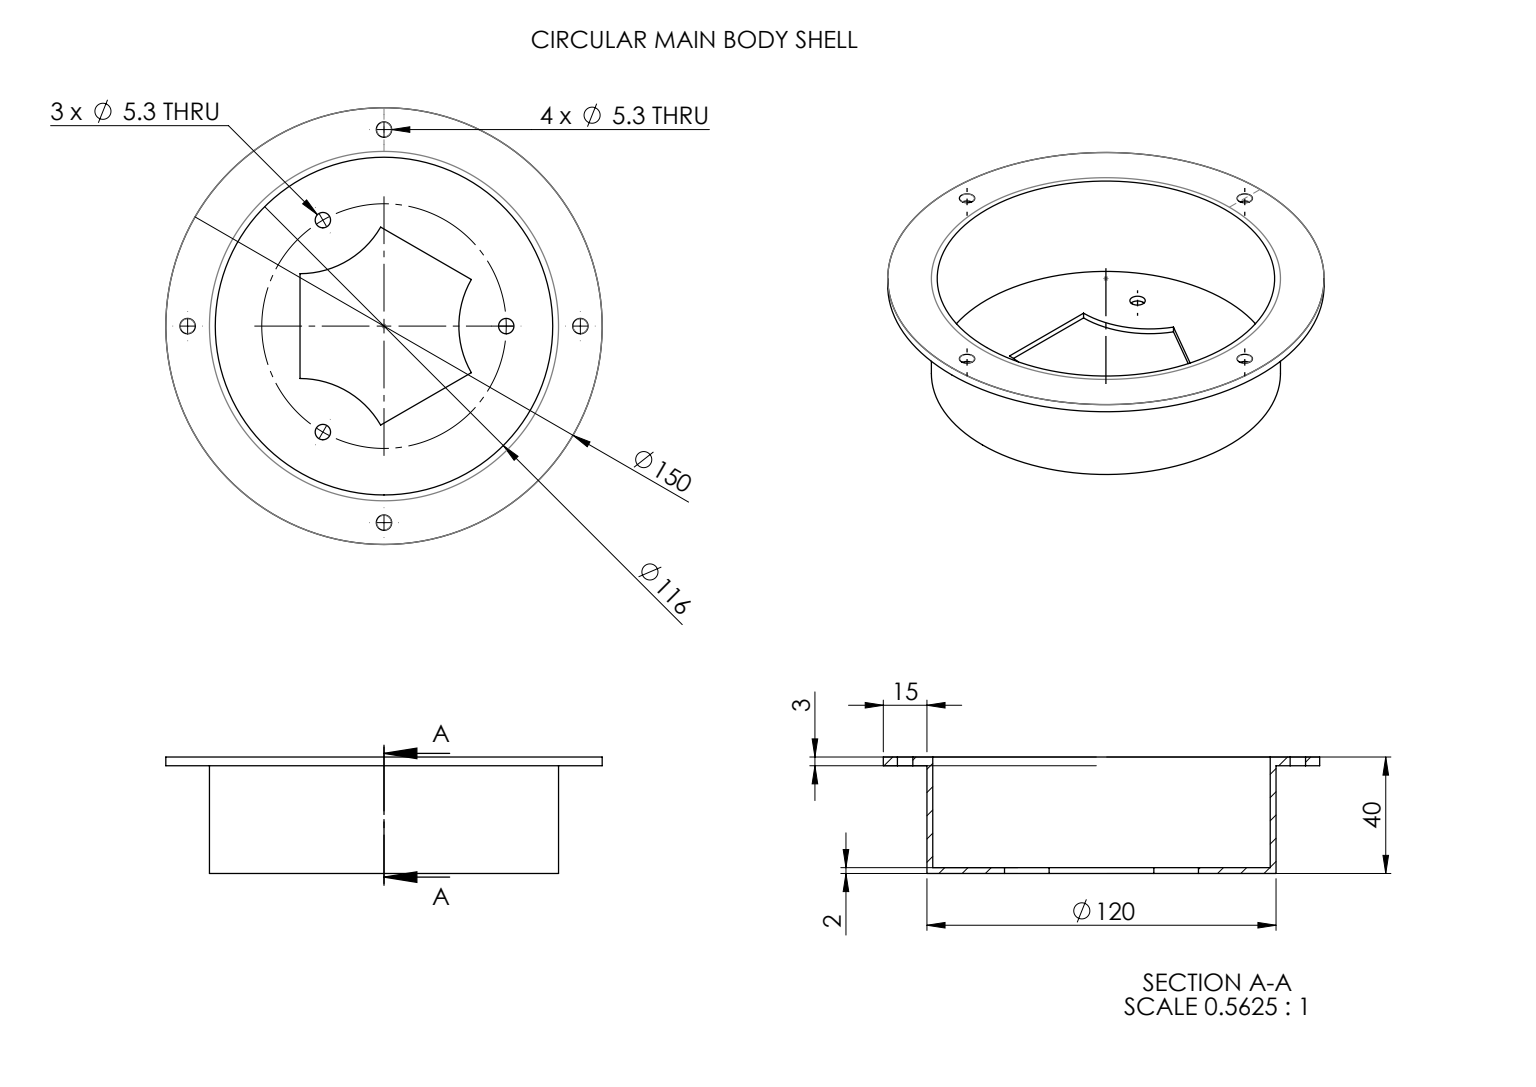
ISO-10303-21;
HEADER;
FILE_DESCRIPTION (('STEP AP214'),
    '1' );
FILE_NAME ('Circular Main Body Shell.step',
    '2026-10-08T13:56:24',
    ( '' ),
    ( '' ),
    'SwSTEP 2.0',
    'SolidWorks 2026',
    '' );
FILE_SCHEMA (( 'AUTOMOTIVE_DESIGN' ));
ENDSEC;

DATA;
#6=VERTEX_POINT ( 'NONE', #1075 ) ;
#10=FACE_OUTER_BOUND ( 'NONE', #8516, .T. ) ;
#19=CYLINDRICAL_SURFACE ( 'NONE', #13536, 2.649999999999992806 ) ;
#21=ADVANCED_FACE ( 'NONE', ( #13423 ), #15876, .F. ) ;
#33=DIRECTION ( 'NONE',  ( 0.000000000000000000, 1.000000000000000000, 0.000000000000000000 ) ) ;
#56=ORIENTED_EDGE ( 'NONE', *, *, #13519, .T. ) ;
#59=VERTEX_POINT ( 'NONE', #6499 ) ;
#76=DIRECTION ( 'NONE',  ( 0.000000000000000000, 1.000000000000000000, 0.000000000000000000 ) ) ;
#81=VECTOR ( 'NONE', #2135, 1000.000000000000000 ) ;
#82=CYLINDRICAL_SURFACE ( 'NONE', #8761, 60.00000000000000000 ) ;
#83=EDGE_CURVE ( 'NONE', #1457, #7914, #2680, .T. ) ;
#86=EDGE_CURVE ( 'NONE', #59, #10154, #4028, .T. ) ;
#101=VECTOR ( 'NONE', #11182, 1000.000000000000000 ) ;
#111=ORIENTED_EDGE ( 'NONE', *, *, #9988, .F. ) ;
#132=DIRECTION ( 'NONE',  ( -0.000000000000000000, -1.000000000000000000, -0.000000000000000000 ) ) ;
#138=VERTEX_POINT ( 'NONE', #361 ) ;
#140=DIRECTION ( 'NONE',  ( 0.000000000000000000, 0.000000000000000000, -1.000000000000000000 ) ) ;
#144=( GEOMETRIC_REPRESENTATION_CONTEXT ( 3 ) GLOBAL_UNCERTAINTY_ASSIGNED_CONTEXT ( ( #8076 ) ) GLOBAL_UNIT_ASSIGNED_CONTEXT ( ( #8304, #5944, #13354 ) ) REPRESENTATION_CONTEXT ( 'NONE', 'WORKASPACE' ) );
#151=DIRECTION ( 'NONE',  ( 0.000000000000000000, 1.000000000000000000, 0.000000000000000000 ) ) ;
#167=VECTOR ( 'NONE', #2072, 1000.000000000000000 ) ;
#187=AXIS2_PLACEMENT_3D ( 'NONE', #15569, #9111, #5544 ) ;
#226=EDGE_CURVE ( 'NONE', #3694, #59, #13994, .T. ) ;
#237=CARTESIAN_POINT ( 'NONE',  ( 0.000000000000000000, 37.00000000000000000, 0.000000000000000000 ) ) ;
#246=ORIENTED_EDGE ( 'NONE', *, *, #2734, .T. ) ;
#248=ORIENTED_EDGE ( 'NONE', *, *, #7361, .F. ) ;
#256=AXIS2_PLACEMENT_3D ( 'NONE', #544, #2863, #5079 ) ;
#267=ORIENTED_EDGE ( 'NONE', *, *, #8923, .F. ) ;
#295=PRODUCT_DEFINITION_CONTEXT ( 'detailed design', #4442, 'design' ) ;
#312=EDGE_CURVE ( 'NONE', #2273, #15957, #6128, .T. ) ;
#325=ORIENTED_EDGE ( 'NONE', *, *, #13615, .F. ) ;
#345=AXIS2_PLACEMENT_3D ( 'NONE', #12427, #14786, #2573 ) ;
#361=CARTESIAN_POINT ( 'NONE',  ( 67.49999999999931788, 40.00000000000000000, 2.650000000000013678 ) ) ;
#364=ADVANCED_FACE ( 'NONE', ( #4243 ), #462, .T. ) ;
#368=CARTESIAN_POINT ( 'NONE',  ( 0.000000000000000000, 40.00000000000000000, 0.000000000000000000 ) ) ;
#377=ORIENTED_EDGE ( 'NONE', *, *, #15710, .F. ) ;
#382=DIRECTION ( 'NONE',  ( -0.000000000000000000, -1.000000000000000000, -0.000000000000000000 ) ) ;
#387=CIRCLE ( 'NONE', #3230, 2.649999999999985700 ) ;
#406=DIRECTION ( 'NONE',  ( -0.000000000000000000, -1.000000000000000000, -0.000000000000000000 ) ) ;
#415=PLANE ( 'NONE',  #1616 ) ;
#434=VERTEX_POINT ( 'NONE', #14346 ) ;
#447=DIRECTION ( 'NONE',  ( 0.000000000000000000, 0.000000000000000000, 1.000000000000000000 ) ) ;
#452=AXIS2_PLACEMENT_3D ( 'NONE', #5371, #14093, #447 ) ;
#460=EDGE_LOOP ( 'NONE', ( #1578, #12472, #3436, #12198 ) ) ;
#462=CYLINDRICAL_SURFACE ( 'NONE', #5357, 75.00000000000001421 ) ;
#515=CARTESIAN_POINT ( 'NONE',  ( 0.000000000000000000, 37.00000000000000000, 75.00000000000001421 ) ) ;
#544=CARTESIAN_POINT ( 'NONE',  ( -67.50000000000000000, 40.00000000000000000, -7.070249711157346244E-13 ) ) ;
#558=EDGE_LOOP ( 'NONE', ( #4178, #10902, #2223, #13257 ) ) ;
#573=DIRECTION ( 'NONE',  ( 0.000000000000000000, 1.000000000000000000, 0.000000000000000000 ) ) ;
#584=DIRECTION ( 'NONE',  ( 0.000000000000000000, 1.000000000000000000, 0.000000000000000000 ) ) ;
#615=VERTEX_POINT ( 'NONE', #3712 ) ;
#631=CARTESIAN_POINT ( 'NONE',  ( 2.143131898507869826E-15, 37.00000000000000000, -67.50000000000000000 ) ) ;
#642=EDGE_LOOP ( 'NONE', ( #4159, #10843 ) ) ;
#646=DIRECTION ( 'NONE',  ( -0.000000000000000000, -1.000000000000000000, -0.000000000000000000 ) ) ;
#660=VECTOR ( 'NONE', #7753, 1000.000000000000000 ) ;
#674=CIRCLE ( 'NONE', #6869, 2.649999999999985700 ) ;
#675=ORIENTED_EDGE ( 'NONE', *, *, #4801, .F. ) ;
#688=EDGE_CURVE ( 'NONE', #4101, #6399, #11429, .T. ) ;
#691=( NAMED_UNIT ( * ) SI_UNIT ( $, .STERADIAN. ) SOLID_ANGLE_UNIT ( ) );
#694=AXIS2_PLACEMENT_3D ( 'NONE', #3412, #1145, #4634 ) ;
#706=DIRECTION ( 'NONE',  ( 0.000000000000000000, 0.000000000000000000, 1.000000000000000000 ) ) ;
#731=CIRCLE ( 'NONE', #9748, 32.00000000000000000 ) ;
#738=EDGE_LOOP ( 'NONE', ( #9185, #775, #5500, #912 ) ) ;
#739=VERTEX_POINT ( 'NONE', #11389 ) ;
#759=VECTOR ( 'NONE', #12567, 1000.000000000000000 ) ;
#760=ORIENTED_EDGE ( 'NONE', *, *, #7226, .T. ) ;
#775=ORIENTED_EDGE ( 'NONE', *, *, #5162, .T. ) ;
#783=FACE_BOUND ( 'NONE', #9056, .T. ) ;
#792=ORIENTED_EDGE ( 'NONE', *, *, #4767, .T. ) ;
#825=CARTESIAN_POINT ( 'NONE',  ( 0.000000000000000000, 37.00000000000000000, 0.000000000000000000 ) ) ;
#826=AXIS2_PLACEMENT_3D ( 'NONE', #2213, #7167, #7316 ) ;
#833=ADVANCED_FACE ( 'NONE', ( #10189, #4033, #2825, #6724, #1611 ), #415, .T. ) ;
#865=VERTEX_POINT ( 'NONE', #5510 ) ;
#881=DIRECTION ( 'NONE',  ( -0.000000000000000000, -1.000000000000000000, -0.000000000000000000 ) ) ;
#896=PLANE ( 'NONE',  #9190 ) ;
#911=( GEOMETRIC_REPRESENTATION_CONTEXT ( 3 ) GLOBAL_UNCERTAINTY_ASSIGNED_CONTEXT ( ( #10140 ) ) GLOBAL_UNIT_ASSIGNED_CONTEXT ( ( #15799, #6830, #4795 ) ) REPRESENTATION_CONTEXT ( 'NONE', 'WORKASPACE' ) );
#912=ORIENTED_EDGE ( 'NONE', *, *, #2834, .T. ) ;
#945=EDGE_LOOP ( 'NONE', ( #10035, #9827 ) ) ;
#946=VERTEX_POINT ( 'NONE', #1706 ) ;
#953=EDGE_CURVE ( 'NONE', #7835, #12023, #11561, .T. ) ;
#956=ADVANCED_FACE ( 'NONE', ( #10366 ), #15296, .F. ) ;
#975=DIRECTION ( 'NONE',  ( -0.000000000000000000, -1.000000000000000000, -0.000000000000000000 ) ) ;
#976=AXIS2_PLACEMENT_3D ( 'NONE', #15540, #4455, #14550 ) ;
#986=AXIS2_PLACEMENT_3D ( 'NONE', #11840, #10645, #6771 ) ;
#989=ORIENTED_EDGE ( 'NONE', *, *, #8609, .T. ) ;
#1007=ORIENTED_EDGE ( 'NONE', *, *, #15616, .T. ) ;
#1038=DIRECTION ( 'NONE',  ( 0.000000000000000000, 1.000000000000000000, 0.000000000000000000 ) ) ;
#1044=LINE ( 'NONE', #14705, #13288 ) ;
#1056=ORIENTED_EDGE ( 'NONE', *, *, #14475, .T. ) ;
#1062=ORIENTED_EDGE ( 'NONE', *, *, #11599, .T. ) ;
#1070=CARTESIAN_POINT ( 'NONE',  ( -1.154700538379255903, 0.000000000000000000, 34.00000000000000000 ) ) ;
#1075=CARTESIAN_POINT ( 'NONE',  ( 42.02221399786069611, -1.230770033143087371E-15, -2.649999999999878231 ) ) ;
#1080=SURFACE_SIDE_STYLE ('',( #10941 ) ) ;
#1120=LINE ( 'NONE', #3465, #2794 ) ;
#1134=CARTESIAN_POINT ( 'NONE',  ( 57.73502691896258199, -20.00000000000000000, 2.081668171172168513E-14 ) ) ;
#1145=DIRECTION ( 'NONE',  ( 0.000000000000000000, 1.000000000000000000, 0.000000000000000000 ) ) ;
#1150=ORIENTED_EDGE ( 'NONE', *, *, #5943, .T. ) ;
#1154=FILL_AREA_STYLE ('',( #15648 ) ) ;
#1161=EDGE_CURVE ( 'NONE', #13011, #10876, #5502, .T. ) ;
#1169=VERTEX_POINT ( 'NONE', #13399 ) ;
#1225=AXIS2_PLACEMENT_3D ( 'NONE', #6934, #1826, #1750 ) ;
#1235=ADVANCED_FACE ( 'NONE', ( #10 ), #1285, .F. ) ;
#1263=FACE_BOUND ( 'NONE', #7017, .T. ) ;
#1275=VERTEX_POINT ( 'NONE', #12264 ) ;
#1281=ORIENTED_EDGE ( 'NONE', *, *, #8662, .T. ) ;
#1285=CYLINDRICAL_SURFACE ( 'NONE', #6526, 2.649999999999992806 ) ;
#1356=DIRECTION ( 'NONE',  ( -0.000000000000000000, -1.000000000000000000, -0.000000000000000000 ) ) ;
#1371=EDGE_LOOP ( 'NONE', ( #10340, #15637, #15181, #9864 ) ) ;
#1374=ORIENTED_EDGE ( 'NONE', *, *, #4282, .F. ) ;
#1383=EDGE_CURVE ( 'NONE', #138, #615, #4026, .T. ) ;
#1387=ORIENTED_EDGE ( 'NONE', *, *, #5738, .T. ) ;
#1457=VERTEX_POINT ( 'NONE', #5415 ) ;
#1471=CARTESIAN_POINT ( 'NONE',  ( 67.49999999999931788, 40.00000000000000000, 2.081668171172168513E-14 ) ) ;
#1478=CIRCLE ( 'NONE', #4839, 60.00000000000000000 ) ;
#1494=CARTESIAN_POINT ( 'NONE',  ( 67.49999999999931788, 37.00000000000000000, -2.649999999999964828 ) ) ;
#1526=EDGE_LOOP ( 'NONE', ( #5441, #6855, #1062, #15045 ) ) ;
#1531=LINE ( 'NONE', #13549, #15735 ) ;
#1533=DIRECTION ( 'NONE',  ( -0.000000000000000000, -1.000000000000000000, -0.000000000000000000 ) ) ;
#1555=ADVANCED_FACE ( 'NONE', ( #7105 ), #2081, .F. ) ;
#1578=ORIENTED_EDGE ( 'NONE', *, *, #15530, .F. ) ;
#1590=CIRCLE ( 'NONE', #826, 2.649999999999985700 ) ;
#1611=FACE_BOUND ( 'NONE', #4354, .T. ) ;
#1616=AXIS2_PLACEMENT_3D ( 'NONE', #5338, #10277, #15205 ) ;
#1618=AXIS2_PLACEMENT_3D ( 'NONE', #10717, #15416, #6844 ) ;
#1635=DIRECTION ( 'NONE',  ( -0.000000000000000000, -1.000000000000000000, -0.000000000000000000 ) ) ;
#1654=VERTEX_POINT ( 'NONE', #7262 ) ;
#1662=AXIS2_PLACEMENT_3D ( 'NONE', #13941, #5063, #2795 ) ;
#1671=ORIENTED_EDGE ( 'NONE', *, *, #6597, .T. ) ;
#1673=( GEOMETRIC_REPRESENTATION_CONTEXT ( 3 ) GLOBAL_UNCERTAINTY_ASSIGNED_CONTEXT ( ( #6941 ) ) GLOBAL_UNIT_ASSIGNED_CONTEXT ( ( #8215, #13115, #691 ) ) REPRESENTATION_CONTEXT ( 'NONE', 'WORKASPACE' ) );
#1706=CARTESIAN_POINT ( 'NONE',  ( -28.86751345948145442, 1.999999999999994893, -18.00000000000001066 ) ) ;
#1713=CIRCLE ( 'NONE', #1979, 57.99999999999999289 ) ;
#1717=EDGE_LOOP ( 'NONE', ( #3204, #14325, #8748, #11994 ) ) ;
#1718=AXIS2_PLACEMENT_3D ( 'NONE', #2231, #7261, #4667 ) ;
#1732=EDGE_CURVE ( 'NONE', #1275, #10154, #13943, .T. ) ;
#1750=DIRECTION ( 'NONE',  ( 0.000000000000000000, 0.000000000000000000, 1.000000000000000000 ) ) ;
#1779=CARTESIAN_POINT ( 'NONE',  ( 0.000000000000000000, 2.000000000000001776, -57.99999999999999289 ) ) ;
#1792=PRODUCT_CONTEXT ( 'NONE', #13090, 'mechanical' ) ;
#1798=ORIENTED_EDGE ( 'NONE', *, *, #688, .F. ) ;
#1811=EDGE_CURVE ( 'NONE', #1275, #3694, #5749, .T. ) ;
#1826=DIRECTION ( 'NONE',  ( 0.000000000000000000, 1.000000000000000000, 0.000000000000000000 ) ) ;
#1838=DIRECTION ( 'NONE',  ( 0.000000000000000000, 0.000000000000000000, -1.000000000000000000 ) ) ;
#1846=CARTESIAN_POINT ( 'NONE',  ( -21.01110699893060030, 2.000000000000000000, 36.39230484541324273 ) ) ;
#1851=EDGE_LOOP ( 'NONE', ( #10259, #13734, #246, #14447 ) ) ;
#1854=DIRECTION ( 'NONE',  ( 9.048317650695024227E-15, 0.000000000000000000, 1.000000000000000000 ) ) ;
#1863=SHAPE_DEFINITION_REPRESENTATION ( #4609, #14733 ) ;
#1889=EDGE_LOOP ( 'NONE', ( #3943, #12784, #12058, #10841 ) ) ;
#1902=PLANE ( 'NONE',  #13101 ) ;
#1931=VECTOR ( 'NONE', #6950, 1000.000000000000000 ) ;
#1933=ADVANCED_FACE ( 'NONE', ( #14354, #11835, #11910, #783, #3283, #4415 ), #5777, .T. ) ;
#1939=VECTOR ( 'NONE', #2696, 1000.000000000000227 ) ;
#1971=EDGE_CURVE ( 'NONE', #2273, #15878, #13430, .T. ) ;
#1979=AXIS2_PLACEMENT_3D ( 'NONE', #2128, #11091, #15945 ) ;
#1989=PRODUCT_DEFINITION_FORMATION_WITH_SPECIFIED_SOURCE ( 'ANY', '', #3575, .NOT_KNOWN. ) ;
#1992=DIRECTION ( 'NONE',  ( -0.000000000000000000, -1.000000000000000000, -0.000000000000000000 ) ) ;
#2010=DIRECTION ( 'NONE',  ( 0.000000000000000000, 0.000000000000000000, 1.000000000000000000 ) ) ;
#2016=ORIENTED_EDGE ( 'NONE', *, *, #6491, .F. ) ;
#2035=CIRCLE ( 'NONE', #4097, 2.649999999999985700 ) ;
#2040=DIRECTION ( 'NONE',  ( 0.000000000000000000, 0.000000000000000000, -1.000000000000000000 ) ) ;
#2044=EDGE_CURVE ( 'NONE', #7914, #615, #1590, .T. ) ;
#2067=FACE_OUTER_BOUND ( 'NONE', #12399, .T. ) ;
#2072=DIRECTION ( 'NONE',  ( -0.000000000000000000, -1.000000000000000000, -0.000000000000000000 ) ) ;
#2075=ORIENTED_EDGE ( 'NONE', *, *, #11616, .F. ) ;
#2078=CARTESIAN_POINT ( 'NONE',  ( 0.000000000000000000, 40.00000000000000000, -57.99999999999999289 ) ) ;
#2081=CYLINDRICAL_SURFACE ( 'NONE', #8849, 2.649999999999992806 ) ;
#2083=ADVANCED_FACE ( 'NONE', ( #12146 ), #6102, .F. ) ;
#2091=DIRECTION ( 'NONE',  ( 0.000000000000000000, 0.000000000000000000, -1.000000000000000000 ) ) ;
#2096=FACE_OUTER_BOUND ( 'NONE', #1526, .T. ) ;
#2128=CARTESIAN_POINT ( 'NONE',  ( 0.000000000000000000, 2.000000000000001776, 0.000000000000000000 ) ) ;
#2131=SURFACE_STYLE_USAGE ( .BOTH. , #1080 ) ;
#2134=CARTESIAN_POINT ( 'NONE',  ( -50.51988060489983212, 0.000000000000000000, 62.50099999999999767 ) ) ;
#2135=DIRECTION ( 'NONE',  ( -0.000000000000000000, -1.000000000000000000, -0.000000000000000000 ) ) ;
#2151=DIRECTION ( 'NONE',  ( -0.000000000000000000, -1.000000000000000000, -0.000000000000000000 ) ) ;
#2164=FACE_BOUND ( 'NONE', #10857, .T. ) ;
#2174=ORIENTED_EDGE ( 'NONE', *, *, #2044, .T. ) ;
#2198=CYLINDRICAL_SURFACE ( 'NONE', #694, 75.00000000000001421 ) ;
#2203=SURFACE_STYLE_FILL_AREA ( #14189 ) ;
#2213=CARTESIAN_POINT ( 'NONE',  ( 67.49999999999931788, 37.00000000000000000, 2.081668171172168513E-14 ) ) ;
#2220=VERTEX_POINT ( 'NONE', #14073 ) ;
#2223=ORIENTED_EDGE ( 'NONE', *, *, #7879, .T. ) ;
#2231=CARTESIAN_POINT ( 'NONE',  ( -21.01110699893060030, 2.000000000000000000, 36.39230484541324273 ) ) ;
#2234=VECTOR ( 'NONE', #10201, 1000.000000000000000 ) ;
#2235=DIRECTION ( 'NONE',  ( -0.000000000000000000, -1.000000000000000000, -0.000000000000000000 ) ) ;
#2250=LINE ( 'NONE', #8497, #12002 ) ;
#2273=VERTEX_POINT ( 'NONE', #5913 ) ;
#2274=CIRCLE ( 'NONE', #11563, 57.99999999999999289 ) ;
#2361=CARTESIAN_POINT ( 'NONE',  ( 42.02221399786069611, 0.000000000000000000, 1.075528555105620399E-13 ) ) ;
#2403=FACE_OUTER_BOUND ( 'NONE', #3347, .T. ) ;
#2484=DIRECTION ( 'NONE',  ( 0.000000000000000000, 0.000000000000000000, 1.000000000000000000 ) ) ;
#2502=AXIS2_PLACEMENT_3D ( 'NONE', #8052, #3348, #14421 ) ;
#2560=ORIENTED_EDGE ( 'NONE', *, *, #5738, .F. ) ;
#2571=DIRECTION ( 'NONE',  ( -0.000000000000000000, -1.000000000000000000, -0.000000000000000000 ) ) ;
#2573=DIRECTION ( 'NONE',  ( 0.000000000000000000, 0.000000000000000000, -1.000000000000000000 ) ) ;
#2596=EDGE_LOOP ( 'NONE', ( #9917, #6295, #11447, #4939 ) ) ;
#2617=DIRECTION ( 'NONE',  ( 0.000000000000000000, 0.000000000000000000, -1.000000000000000000 ) ) ;
#2668=CARTESIAN_POINT ( 'NONE',  ( 9.184850993605150311E-15, 37.00000000000000000, -75.00000000000001421 ) ) ;
#2673=DIRECTION ( 'NONE',  ( 0.000000000000000000, 0.000000000000000000, 1.000000000000000000 ) ) ;
#2676=DIRECTION ( 'NONE',  ( -0.000000000000000000, -1.000000000000000000, -0.000000000000000000 ) ) ;
#2680=LINE ( 'NONE', #15061, #6377 ) ;
#2685=CIRCLE ( 'NONE', #8936, 2.649999999999985700 ) ;
#2686=CIRCLE ( 'NONE', #10444, 2.649999999999985700 ) ;
#2696=DIRECTION ( 'NONE',  ( -0.8660254037844408170, -0.000000000000000000, -0.4999999999999961142 ) ) ;
#2702=ORIENTED_EDGE ( 'NONE', *, *, #8509, .T. ) ;
#2731=EDGE_CURVE ( 'NONE', #15878, #1169, #11203, .T. ) ;
#2734=EDGE_CURVE ( 'NONE', #615, #7914, #2686, .T. ) ;
#2745=ORIENTED_EDGE ( 'NONE', *, *, #6491, .T. ) ;
#2772=EDGE_CURVE ( 'NONE', #7134, #5346, #13221, .T. ) ;
#2792=AXIS2_PLACEMENT_3D ( 'NONE', #14224, #4368, #9302 ) ;
#2793=FACE_OUTER_BOUND ( 'NONE', #15403, .T. ) ;
#2794=VECTOR ( 'NONE', #975, 1000.000000000000000 ) ;
#2795=DIRECTION ( 'NONE',  ( 0.000000000000000000, 0.000000000000000000, 1.000000000000000000 ) ) ;
#2825=FACE_BOUND ( 'NONE', #13224, .T. ) ;
#2834=EDGE_CURVE ( 'NONE', #434, #10287, #5541, .T. ) ;
#2849=AXIS2_PLACEMENT_3D ( 'NONE', #10462, #4319, #9259 ) ;
#2863=DIRECTION ( 'NONE',  ( 0.000000000000000000, 1.000000000000000000, 0.000000000000000000 ) ) ;
#2924=EDGE_LOOP ( 'NONE', ( #7893, #9587, #3567, #3170 ) ) ;
#2973=CARTESIAN_POINT ( 'NONE',  ( 67.49999999999931788, 37.00000000000000000, 2.650000000000013678 ) ) ;
#2986=ORIENTED_EDGE ( 'NONE', *, *, #3942, .F. ) ;
#2996=DIRECTION ( 'NONE',  ( 0.4999999999999998890, 0.000000000000000000, 0.8660254037844387076 ) ) ;
#3012=VECTOR ( 'NONE', #7245, 1000.000000000000000 ) ;
#3032=CARTESIAN_POINT ( 'NONE',  ( -6.765421556309547668E-13, 40.00000000000000000, 67.49999999999930367 ) ) ;
#3035=EDGE_CURVE ( 'NONE', #5346, #10287, #3930, .T. ) ;
#3043=CIRCLE ( 'NONE', #14152, 75.00000000000001421 ) ;
#3044=CARTESIAN_POINT ( 'NONE',  ( 0.000000000000000000, 0.000000000000000000, 0.000000000000000000 ) ) ;
#3079=ORIENTED_EDGE ( 'NONE', *, *, #14190, .T. ) ;
#3087=CIRCLE ( 'NONE', #256, 2.649999999999992806 ) ;
#3100=ORIENTED_EDGE ( 'NONE', *, *, #5391, .T. ) ;
#3112=ORIENTED_EDGE ( 'NONE', *, *, #5162, .F. ) ;
#3120=FACE_OUTER_BOUND ( 'NONE', #4526, .T. ) ;
#3122=CARTESIAN_POINT ( 'NONE',  ( -28.86751345948126257, -20.00000000000000000, -50.00000000000000711 ) ) ;
#3125=LINE ( 'NONE', #10644, #10930 ) ;
#3145=DIRECTION ( 'NONE',  ( 0.000000000000000000, 1.000000000000000000, 0.000000000000000000 ) ) ;
#3170=ORIENTED_EDGE ( 'NONE', *, *, #7879, .F. ) ;
#3192=ORIENTED_EDGE ( 'NONE', *, *, #4801, .T. ) ;
#3200=DIRECTION ( 'NONE',  ( -0.000000000000000000, -1.000000000000000000, -0.000000000000000000 ) ) ;
#3204=ORIENTED_EDGE ( 'NONE', *, *, #8662, .F. ) ;
#3223=AXIS2_PLACEMENT_3D ( 'NONE', #11897, #11972, #4638 ) ;
#3227=PLANE ( 'NONE',  #6600 ) ;
#3230=AXIS2_PLACEMENT_3D ( 'NONE', #10329, #7502, #11515 ) ;
#3235=EDGE_CURVE ( 'NONE', #15957, #1169, #3125, .T. ) ;
#3254=ADVANCED_FACE ( 'NONE', ( #5867 ), #15574, .F. ) ;
#3268=SURFACE_STYLE_USAGE ( .BOTH. , #7154 ) ;
#3279=ADVANCED_FACE ( 'NONE', ( #2067 ), #1902, .F. ) ;
#3282=AXIS2_PLACEMENT_3D ( 'NONE', #11517, #7666, #12565 ) ;
#3283=FACE_BOUND ( 'NONE', #12989, .T. ) ;
#3286=DIRECTION ( 'NONE',  ( -0.000000000000000000, -1.000000000000000000, -0.000000000000000000 ) ) ;
#3333=EDGE_LOOP ( 'NONE', ( #12994, #325 ) ) ;
#3346=EDGE_CURVE ( 'NONE', #7037, #1654, #14509, .T. ) ;
#3347=EDGE_LOOP ( 'NONE', ( #5791, #8130, #7271, #13989 ) ) ;
#3348=DIRECTION ( 'NONE',  ( 0.000000000000000000, 1.000000000000000000, 0.000000000000000000 ) ) ;
#3361=DIRECTION ( 'NONE',  ( 0.000000000000000000, 0.000000000000000000, -1.000000000000000000 ) ) ;
#3391=ORIENTED_EDGE ( 'NONE', *, *, #83, .T. ) ;
#3412=CARTESIAN_POINT ( 'NONE',  ( 0.000000000000000000, 37.00000000000000000, 0.000000000000000000 ) ) ;
#3429=CARTESIAN_POINT ( 'NONE',  ( 0.000000000000000000, 40.00000000000000000, -57.99999999999999289 ) ) ;
#3436=ORIENTED_EDGE ( 'NONE', *, *, #3346, .T. ) ;
#3442=FACE_OUTER_BOUND ( 'NONE', #11276, .T. ) ;
#3465=CARTESIAN_POINT ( 'NONE',  ( 42.02221399786069611, 0.000000000000000000, -2.649999999999884892 ) ) ;
#3467=CARTESIAN_POINT ( 'NONE',  ( -21.01110699893060030, 0.000000000000000000, 36.39230484541324273 ) ) ;
#3480=EDGE_CURVE ( 'NONE', #11871, #12864, #13849, .T. ) ;
#3500=AXIS2_PLACEMENT_3D ( 'NONE', #5960, #2151, #8629 ) ;
#3527=VECTOR ( 'NONE', #1635, 1000.000000000000000 ) ;
#3548=AXIS2_PLACEMENT_3D ( 'NONE', #10049, #6414, #2673 ) ;
#3567=ORIENTED_EDGE ( 'NONE', *, *, #12620, .F. ) ;
#3575=PRODUCT ( 'Circular Main Body Shell', 'Circular Main Body Shell', '', ( #1792 ) ) ;
#3577=FACE_OUTER_BOUND ( 'NONE', #13494, .T. ) ;
#3608=FACE_BOUND ( 'NONE', #15163, .T. ) ;
#3665=ADVANCED_FACE ( 'NONE', ( #15396 ), #5528, .F. ) ;
#3678=ORIENTED_EDGE ( 'NONE', *, *, #7728, .T. ) ;
#3694=VERTEX_POINT ( 'NONE', #8048 ) ;
#3695=CARTESIAN_POINT ( 'NONE',  ( 79.38739406438118351, 1.999999999999998224, 12.50099999999964417 ) ) ;
#3705=DIRECTION ( 'NONE',  ( -0.000000000000000000, -1.000000000000000000, -0.000000000000000000 ) ) ;
#3712=CARTESIAN_POINT ( 'NONE',  ( 67.49999999999931788, 37.00000000000000000, 2.650000000000006573 ) ) ;
#3755=ADVANCED_FACE ( 'NONE', ( #3577 ), #2198, .T. ) ;
#3766=DIRECTION ( 'NONE',  ( 0.000000000000000000, -0.000000000000000000, 1.000000000000000000 ) ) ;
#3773=DIRECTION ( 'NONE',  ( 0.000000000000000000, 0.000000000000000000, 1.000000000000000000 ) ) ;
#3894=EDGE_LOOP ( 'NONE', ( #8906, #760 ) ) ;
#3924=ADVANCED_FACE ( 'NONE', ( #5112 ), #8837, .T. ) ;
#3930=LINE ( 'NONE', #12806, #4979 ) ;
#3937=ORIENTED_EDGE ( 'NONE', *, *, #7399, .F. ) ;
#3942=EDGE_CURVE ( 'NONE', #138, #1457, #7143, .T. ) ;
#3943=ORIENTED_EDGE ( 'NONE', *, *, #6047, .T. ) ;
#3995=EDGE_LOOP ( 'NONE', ( #1798, #13792, #7346, #5691 ) ) ;
#4004=CARTESIAN_POINT ( 'NONE',  ( -50.51988060489983212, 1.999999999999998224, 62.50099999999999767 ) ) ;
#4017=VECTOR ( 'NONE', #1356, 1000.000000000000000 ) ;
#4026=LINE ( 'NONE', #2973, #9618 ) ;
#4028=CIRCLE ( 'NONE', #12800, 60.00000000000000000 ) ;
#4033=FACE_BOUND ( 'NONE', #11763, .T. ) ;
#4038=ORIENTED_EDGE ( 'NONE', *, *, #3942, .T. ) ;
#4042=VERTEX_POINT ( 'NONE', #8037 ) ;
#4057=ORIENTED_EDGE ( 'NONE', *, *, #3235, .F. ) ;
#4097=AXIS2_PLACEMENT_3D ( 'NONE', #11691, #4188, #1838 ) ;
#4101=VERTEX_POINT ( 'NONE', #8943 ) ;
#4106=ORIENTED_EDGE ( 'NONE', *, *, #226, .F. ) ;
#4110=CIRCLE ( 'NONE', #5926, 57.99999999999999289 ) ;
#4154=CARTESIAN_POINT ( 'NONE',  ( 2.143131898507869826E-15, 37.00000000000000000, -67.50000000000000000 ) ) ;
#4159=ORIENTED_EDGE ( 'NONE', *, *, #12723, .F. ) ;
#4167=DIRECTION ( 'NONE',  ( -0.000000000000000000, -1.000000000000000000, -0.000000000000000000 ) ) ;
#4178=ORIENTED_EDGE ( 'NONE', *, *, #13550, .F. ) ;
#4187=DIRECTION ( 'NONE',  ( 0.000000000000000000, 0.000000000000000000, -1.000000000000000000 ) ) ;
#4188=DIRECTION ( 'NONE',  ( -0.000000000000000000, -1.000000000000000000, -0.000000000000000000 ) ) ;
#4209=CARTESIAN_POINT ( 'NONE',  ( -50.51988060489983212, 1.999999999999998224, 62.50099999999999767 ) ) ;
#4225=CARTESIAN_POINT ( 'NONE',  ( 42.02221399786069611, 2.000000000000000000, 1.075528555105620399E-13 ) ) ;
#4243=FACE_OUTER_BOUND ( 'NONE', #6518, .T. ) ;
#4279=DIRECTION ( 'NONE',  ( 8.673617379884035472E-16, 0.000000000000000000, 1.000000000000000000 ) ) ;
#4282=EDGE_CURVE ( 'NONE', #14880, #10728, #7157, .T. ) ;
#4319=DIRECTION ( 'NONE',  ( -0.000000000000000000, -1.000000000000000000, -0.000000000000000000 ) ) ;
#4323=ORIENTED_EDGE ( 'NONE', *, *, #15530, .T. ) ;
#4326=CARTESIAN_POINT ( 'NONE',  ( -1.154700538379235031, 1.999999999999998224, -34.00000000000000000 ) ) ;
#4354=EDGE_LOOP ( 'NONE', ( #2016, #3937, #6611, #9493, #248, #8433 ) ) ;
#4367=DIRECTION ( 'NONE',  ( -0.000000000000000000, -1.000000000000000000, -0.000000000000000000 ) ) ;
#4368=DIRECTION ( 'NONE',  ( -0.000000000000000000, -1.000000000000000000, -0.000000000000000000 ) ) ;
#4375=ORIENTED_EDGE ( 'NONE', *, *, #9521, .T. ) ;
#4385=FACE_OUTER_BOUND ( 'NONE', #14907, .T. ) ;
#4412=DIRECTION ( 'NONE',  ( 0.000000000000000000, 1.000000000000000000, 0.000000000000000000 ) ) ;
#4415=FACE_OUTER_BOUND ( 'NONE', #6444, .T. ) ;
#4442=APPLICATION_CONTEXT ( 'automotive_design' ) ;
#4444=FACE_BOUND ( 'NONE', #945, .T. ) ;
#4455=DIRECTION ( 'NONE',  ( -0.000000000000000000, -1.000000000000000000, -0.000000000000000000 ) ) ;
#4467=AXIS2_PLACEMENT_3D ( 'NONE', #11083, #8823, #14055 ) ;
#4498=EDGE_LOOP ( 'NONE', ( #14987, #11958 ) ) ;
#4513=CARTESIAN_POINT ( 'NONE',  ( 67.49999999999931788, 37.00000000000000000, 2.081668171172168513E-14 ) ) ;
#4519=FACE_BOUND ( 'NONE', #8353, .T. ) ;
#4526=EDGE_LOOP ( 'NONE', ( #14542, #13389, #13917, #11725 ) ) ;
#4538=VECTOR ( 'NONE', #14752, 1000.000000000000000 ) ;
#4545=ADVANCED_FACE ( 'NONE', ( #11286 ), #9040, .F. ) ;
#4566=PRESENTATION_STYLE_ASSIGNMENT (( #2131 ) ) ;
#4579=ORIENTED_EDGE ( 'NONE', *, *, #12723, .T. ) ;
#4609=PRODUCT_DEFINITION_SHAPE ( 'NONE', 'NONE',  #4824 ) ;
#4634=DIRECTION ( 'NONE',  ( 0.000000000000000000, 0.000000000000000000, 1.000000000000000000 ) ) ;
#4638=DIRECTION ( 'NONE',  ( 1.000000000000000000, 0.000000000000000000, 0.000000000000000000 ) ) ;
#4650=LINE ( 'NONE', #3429, #13624 ) ;
#4667=DIRECTION ( 'NONE',  ( 0.000000000000000000, 0.000000000000000000, 1.000000000000000000 ) ) ;
#4682=ORIENTED_EDGE ( 'NONE', *, *, #8054, .T. ) ;
#4704=ADVANCED_FACE ( 'NONE', ( #7007 ), #9276, .T. ) ;
#4712=ORIENTED_EDGE ( 'NONE', *, *, #1811, .F. ) ;
#4751=CARTESIAN_POINT ( 'NONE',  ( 42.02221399786069611, 2.000000000000000000, -2.649999999999884892 ) ) ;
#4767=EDGE_CURVE ( 'NONE', #6399, #5167, #10716, .T. ) ;
#4795=( NAMED_UNIT ( * ) SI_UNIT ( $, .STERADIAN. ) SOLID_ANGLE_UNIT ( ) );
#4798=DIRECTION ( 'NONE',  ( -0.000000000000000000, -1.000000000000000000, -0.000000000000000000 ) ) ;
#4801=EDGE_CURVE ( 'NONE', #7835, #8282, #14633, .T. ) ;
#4803=VECTOR ( 'NONE', #13537, 1000.000000000000227 ) ;
#4824=PRODUCT_DEFINITION ( 'UNKNOWN', '', #1989, #295 ) ;
#4830=LINE ( 'NONE', #11929, #7736 ) ;
#4839=AXIS2_PLACEMENT_3D ( 'NONE', #3044, #7990, #706 ) ;
#4848=CIRCLE ( 'NONE', #2502, 2.649999999999992806 ) ;
#4868=ORIENTED_EDGE ( 'NONE', *, *, #15495, .F. ) ;
#4889=CARTESIAN_POINT ( 'NONE',  ( 0.000000000000000000, 37.00000000000000000, 0.000000000000000000 ) ) ;
#4890=DIRECTION ( 'NONE',  ( 0.000000000000000000, 0.000000000000000000, -1.000000000000000000 ) ) ;
#4908=CARTESIAN_POINT ( 'NONE',  ( -28.86751345948126257, 1.999999999999998224, -50.00000000000000711 ) ) ;
#4932=ADVANCED_FACE ( 'NONE', ( #9645 ), #14667, .F. ) ;
#4939=ORIENTED_EDGE ( 'NONE', *, *, #8923, .T. ) ;
#4979=VECTOR ( 'NONE', #12485, 1000.000000000000000 ) ;
#5016=DIRECTION ( 'NONE',  ( 0.000000000000000000, 1.000000000000000000, -0.000000000000000000 ) ) ;
#5055=ORIENTED_EDGE ( 'NONE', *, *, #8996, .F. ) ;
#5063=DIRECTION ( 'NONE',  ( 0.000000000000000000, 1.000000000000000000, 0.000000000000000000 ) ) ;
#5076=DIRECTION ( 'NONE',  ( -0.000000000000000000, -1.000000000000000000, 0.000000000000000000 ) ) ;
#5079=DIRECTION ( 'NONE',  ( 0.000000000000000000, 0.000000000000000000, 1.000000000000000000 ) ) ;
#5098=DIRECTION ( 'NONE',  ( -0.000000000000000000, -1.000000000000000000, -0.000000000000000000 ) ) ;
#5112=FACE_OUTER_BOUND ( 'NONE', #3995, .T. ) ;
#5140=LINE ( 'NONE', #14007, #1939 ) ;
#5155=DIRECTION ( 'NONE',  ( 0.000000000000000000, 1.000000000000000000, 0.000000000000000000 ) ) ;
#5162=EDGE_CURVE ( 'NONE', #5346, #7134, #7418, .T. ) ;
#5165=CARTESIAN_POINT ( 'NONE',  ( -1.154700538379261232, -20.00000000000000000, 34.00000000000000000 ) ) ;
#5167=VERTEX_POINT ( 'NONE', #11497 ) ;
#5265=DIRECTION ( 'NONE',  ( 0.000000000000000000, 0.000000000000000000, 1.000000000000000000 ) ) ;
#5282=DIRECTION ( 'NONE',  ( -0.000000000000000000, -1.000000000000000000, -0.000000000000000000 ) ) ;
#5283=DIRECTION ( 'NONE',  ( -0.000000000000000000, -1.000000000000000000, -0.000000000000000000 ) ) ;
#5291=AXIS2_PLACEMENT_3D ( 'NONE', #4225, #6747, #9253 ) ;
#5292=DIRECTION ( 'NONE',  ( -0.000000000000000000, -1.000000000000000000, -0.000000000000000000 ) ) ;
#5338=CARTESIAN_POINT ( 'NONE',  ( 0.000000000000000000, 2.000000000000000000, 0.000000000000000000 ) ) ;
#5341=CARTESIAN_POINT ( 'NONE',  ( -21.01110699893060030, 2.000000000000000000, 39.04230484541323420 ) ) ;
#5342=ORIENTED_EDGE ( 'NONE', *, *, #9521, .F. ) ;
#5344=ORIENTED_EDGE ( 'NONE', *, *, #13132, .F. ) ;
#5346=VERTEX_POINT ( 'NONE', #6769 ) ;
#5357=AXIS2_PLACEMENT_3D ( 'NONE', #15080, #12560, #9110 ) ;
#5371=CARTESIAN_POINT ( 'NONE',  ( -21.01110699893041556, 2.000000000000000000, -36.39230484541334221 ) ) ;
#5391=EDGE_CURVE ( 'NONE', #10154, #59, #1478, .T. ) ;
#5415=CARTESIAN_POINT ( 'NONE',  ( 67.49999999999931788, 40.00000000000000000, -2.649999999999971934 ) ) ;
#5434=DIRECTION ( 'NONE',  ( 0.000000000000000000, 1.000000000000000000, 0.000000000000000000 ) ) ;
#5441=ORIENTED_EDGE ( 'NONE', *, *, #15616, .F. ) ;
#5478=ORIENTED_EDGE ( 'NONE', *, *, #953, .T. ) ;
#5494=DIRECTION ( 'NONE',  ( -0.000000000000000000, -1.000000000000000000, -0.000000000000000000 ) ) ;
#5500=ORIENTED_EDGE ( 'NONE', *, *, #15495, .T. ) ;
#5502=CIRCLE ( 'NONE', #345, 2.649999999999985700 ) ;
#5510=CARTESIAN_POINT ( 'NONE',  ( -21.01110699893060030, -1.230770033143087371E-15, 33.74230484541325126 ) ) ;
#5525=CARTESIAN_POINT ( 'NONE',  ( 0.000000000000000000, 40.00000000000000000, 0.000000000000000000 ) ) ;
#5528=CYLINDRICAL_SURFACE ( 'NONE', #2849, 2.649999999999992806 ) ;
#5541=CIRCLE ( 'NONE', #7615, 2.649999999999992806 ) ;
#5544=DIRECTION ( 'NONE',  ( 0.000000000000000000, 0.000000000000000000, -1.000000000000000000 ) ) ;
#5619=ORIENTED_EDGE ( 'NONE', *, *, #12684, .F. ) ;
#5626=AXIS2_PLACEMENT_3D ( 'NONE', #1846, #10424, #2010 ) ;
#5631=DIRECTION ( 'NONE',  ( 0.000000000000000000, 0.000000000000000000, 1.000000000000000000 ) ) ;
#5691=ORIENTED_EDGE ( 'NONE', *, *, #15137, .T. ) ;
#5712=ORIENTED_EDGE ( 'NONE', *, *, #312, .F. ) ;
#5718=EDGE_CURVE ( 'NONE', #7037, #7701, #7960, .T. ) ;
#5731=FACE_OUTER_BOUND ( 'NONE', #4498, .T. ) ;
#5738=EDGE_CURVE ( 'NONE', #8282, #7835, #3043, .T. ) ;
#5749=CIRCLE ( 'NONE', #14782, 60.00000000000000000 ) ;
#5757=FACE_OUTER_BOUND ( 'NONE', #558, .T. ) ;
#5777=PLANE ( 'NONE',  #1618 ) ;
#5780=DIRECTION ( 'NONE',  ( 0.4999999999999961697, 0.000000000000000000, -0.8660254037844409281 ) ) ;
#5791=ORIENTED_EDGE ( 'NONE', *, *, #312, .T. ) ;
#5799=DIRECTION ( 'NONE',  ( 3.111660235033397726E-14, 0.000000000000000000, 1.000000000000000000 ) ) ;
#5851=PRESENTATION_STYLE_ASSIGNMENT (( #3268 ) ) ;
#5855=ORIENTED_EDGE ( 'NONE', *, *, #4282, .T. ) ;
#5867=FACE_OUTER_BOUND ( 'NONE', #9225, .T. ) ;
#5876=ORIENTED_EDGE ( 'NONE', *, *, #11616, .T. ) ;
#5878=FACE_OUTER_BOUND ( 'NONE', #738, .T. ) ;
#5880=ADVANCED_FACE ( 'NONE', ( #10319 ), #11187, .F. ) ;
#5887=AXIS2_PLACEMENT_3D ( 'NONE', #10251, #151, #3773 ) ;
#5893=ORIENTED_EDGE ( 'NONE', *, *, #3480, .T. ) ;
#5913=CARTESIAN_POINT ( 'NONE',  ( -6.765421556309547668E-13, 40.00000000000000000, 64.84999999999931219 ) ) ;
#5916=CARTESIAN_POINT ( 'NONE',  ( 2.143131898507869826E-15, 40.00000000000000000, -67.50000000000000000 ) ) ;
#5926=AXIS2_PLACEMENT_3D ( 'NONE', #6222, #76, #6685 ) ;
#5933=ORIENTED_EDGE ( 'NONE', *, *, #13519, .F. ) ;
#5943=EDGE_CURVE ( 'NONE', #10287, #434, #7175, .T. ) ;
#5944=( NAMED_UNIT ( * ) PLANE_ANGLE_UNIT ( ) SI_UNIT ( $, .RADIAN. ) );
#5949=CARTESIAN_POINT ( 'NONE',  ( 2.143131898507869826E-15, 37.00000000000000000, -70.15000000000000568 ) ) ;
#5960=CARTESIAN_POINT ( 'NONE',  ( -21.01110699893041556, 0.000000000000000000, -36.39230484541334221 ) ) ;
#5978=DIRECTION ( 'NONE',  ( -0.000000000000000000, -1.000000000000000000, -0.000000000000000000 ) ) ;
#5982=CARTESIAN_POINT ( 'NONE',  ( 57.73502691896258199, 0.000000000000000000, 2.081668171172168513E-14 ) ) ;
#5994=EDGE_LOOP ( 'NONE', ( #9149, #1374 ) ) ;
#6012=ORIENTED_EDGE ( 'NONE', *, *, #3346, .F. ) ;
#6038=CARTESIAN_POINT ( 'NONE',  ( 0.000000000000000000, 40.00000000000000000, 75.00000000000001421 ) ) ;
#6047=EDGE_CURVE ( 'NONE', #13808, #739, #4848, .T. ) ;
#6051=ORIENTED_EDGE ( 'NONE', *, *, #1383, .F. ) ;
#6100=AXIS2_PLACEMENT_3D ( 'NONE', #2361, #4798, #8602 ) ;
#6102=CYLINDRICAL_SURFACE ( 'NONE', #15029, 2.649999999999992806 ) ;
#6123=AXIS2_PLACEMENT_3D ( 'NONE', #3122, #6843, #14273 ) ;
#6128=CIRCLE ( 'NONE', #6401, 2.649999999999999467 ) ;
#6148=DIRECTION ( 'NONE',  ( 0.000000000000000000, 0.000000000000000000, -1.000000000000000000 ) ) ;
#6149=CIRCLE ( 'NONE', #1225, 2.649999999999999467 ) ;
#6168=CIRCLE ( 'NONE', #13634, 60.00000000000000000 ) ;
#6201=ORIENTED_EDGE ( 'NONE', *, *, #8996, .T. ) ;
#6222=CARTESIAN_POINT ( 'NONE',  ( 0.000000000000000000, 40.00000000000000000, 0.000000000000000000 ) ) ;
#6263=FACE_OUTER_BOUND ( 'NONE', #13751, .T. ) ;
#6282=CYLINDRICAL_SURFACE ( 'NONE', #11013, 60.00000000000000000 ) ;
#6295=ORIENTED_EDGE ( 'NONE', *, *, #12437, .T. ) ;
#6305=DIRECTION ( 'NONE',  ( 0.000000000000000000, 0.000000000000000000, -1.000000000000000000 ) ) ;
#6335=ORIENTED_EDGE ( 'NONE', *, *, #2731, .F. ) ;
#6366=EDGE_CURVE ( 'NONE', #11846, #13350, #2274, .T. ) ;
#6377=VECTOR ( 'NONE', #7724, 1000.000000000000000 ) ;
#6378=LINE ( 'NONE', #5165, #11998 ) ;
#6399=VERTEX_POINT ( 'NONE', #1070 ) ;
#6401=AXIS2_PLACEMENT_3D ( 'NONE', #3032, #13771, #10240 ) ;
#6414=DIRECTION ( 'NONE',  ( 0.000000000000000000, 1.000000000000000000, 0.000000000000000000 ) ) ;
#6415=CIRCLE ( 'NONE', #2792, 31.99999999999999289 ) ;
#6418=DIRECTION ( 'NONE',  ( 0.000000000000000000, 0.000000000000000000, 1.000000000000000000 ) ) ;
#6444=EDGE_LOOP ( 'NONE', ( #2702, #4375 ) ) ;
#6474=CARTESIAN_POINT ( 'NONE',  ( -1.154700538379252350, 1.999999999999994893, 34.00000000000000000 ) ) ;
#6491=EDGE_CURVE ( 'NONE', #2220, #11871, #12583, .T. ) ;
#6499=CARTESIAN_POINT ( 'NONE',  ( 7.347880794884118356E-15, 0.000000000000000000, 60.00000000000000000 ) ) ;
#6500=EDGE_LOOP ( 'NONE', ( #11006, #3678 ) ) ;
#6518=EDGE_LOOP ( 'NONE', ( #3192, #11357, #8624, #6881 ) ) ;
#6526=AXIS2_PLACEMENT_3D ( 'NONE', #3467, #13552, #8425 ) ;
#6540=DIRECTION ( 'NONE',  ( -0.000000000000000000, -1.000000000000000000, -0.000000000000000000 ) ) ;
#6555=EDGE_LOOP ( 'NONE', ( #12250, #9807 ) ) ;
#6560=LINE ( 'NONE', #9153, #8706 ) ;
#6597=EDGE_CURVE ( 'NONE', #5167, #12864, #7453, .T. ) ;
#6600=AXIS2_PLACEMENT_3D ( 'NONE', #11937, #1038, #8176 ) ;
#6611=ORIENTED_EDGE ( 'NONE', *, *, #8695, .F. ) ;
#6685=DIRECTION ( 'NONE',  ( 0.000000000000000000, 0.000000000000000000, 1.000000000000000000 ) ) ;
#6724=FACE_OUTER_BOUND ( 'NONE', #6500, .T. ) ;
#6747=DIRECTION ( 'NONE',  ( 0.000000000000000000, 1.000000000000000000, 0.000000000000000000 ) ) ;
#6769=CARTESIAN_POINT ( 'NONE',  ( -21.01110699893041556, 2.000000000000000000, -33.74230484541335073 ) ) ;
#6771=DIRECTION ( 'NONE',  ( 0.000000000000000000, 0.000000000000000000, -1.000000000000000000 ) ) ;
#6777=ORIENTED_EDGE ( 'NONE', *, *, #2731, .T. ) ;
#6803=ADVANCED_FACE ( 'NONE', ( #6263 ), #9972, .F. ) ;
#6808=DIRECTION ( 'NONE',  ( -0.000000000000000000, -1.000000000000000000, -0.000000000000000000 ) ) ;
#6830=( NAMED_UNIT ( * ) PLANE_ANGLE_UNIT ( ) SI_UNIT ( $, .RADIAN. ) );
#6843=DIRECTION ( 'NONE',  ( 0.000000000000000000, -1.000000000000000000, 0.000000000000000000 ) ) ;
#6844=DIRECTION ( 'NONE',  ( 0.000000000000000000, -0.000000000000000000, 1.000000000000000000 ) ) ;
#6845=MECHANICAL_DESIGN_GEOMETRIC_PRESENTATION_REPRESENTATION('',(#7352),#144);
#6848=CARTESIAN_POINT ( 'NONE',  ( 79.38739406438118351, 1.999999999999998224, 12.50099999999964417 ) ) ;
#6855=ORIENTED_EDGE ( 'NONE', *, *, #7326, .F. ) ;
#6869=AXIS2_PLACEMENT_3D ( 'NONE', #7114, #13157, #2091 ) ;
#6881=ORIENTED_EDGE ( 'NONE', *, *, #953, .F. ) ;
#6934=CARTESIAN_POINT ( 'NONE',  ( -6.765421556309547668E-13, 40.00000000000000000, 67.49999999999930367 ) ) ;
#6941=UNCERTAINTY_MEASURE_WITH_UNIT (LENGTH_MEASURE( 1.000000000000000082E-05 ), #8215, 'distance_accuracy_value', 'NONE');
#6943=LINE ( 'NONE', #13053, #9701 ) ;
#6950=DIRECTION ( 'NONE',  ( -0.000000000000000000, 1.000000000000000000, 0.000000000000000000 ) ) ;
#6958=DIRECTION ( 'NONE',  ( -0.000000000000000000, -1.000000000000000000, -0.000000000000000000 ) ) ;
#7001=ORIENTED_EDGE ( 'NONE', *, *, #10395, .F. ) ;
#7007=FACE_OUTER_BOUND ( 'NONE', #1717, .T. ) ;
#7017=EDGE_LOOP ( 'NONE', ( #6335, #5344 ) ) ;
#7025=ADVANCED_FACE ( 'NONE', ( #5757 ), #11653, .F. ) ;
#7037=VERTEX_POINT ( 'NONE', #14180 ) ;
#7083=CARTESIAN_POINT ( 'NONE',  ( 0.000000000000000000, 37.00000000000000000, 75.00000000000001421 ) ) ;
#7092=LINE ( 'NONE', #11993, #167 ) ;
#7105=FACE_OUTER_BOUND ( 'NONE', #1889, .T. ) ;
#7114=CARTESIAN_POINT ( 'NONE',  ( 2.143131898507869826E-15, 37.00000000000000000, -67.50000000000000000 ) ) ;
#7132=DIRECTION ( 'NONE',  ( 0.000000000000000000, 1.000000000000000000, 0.000000000000000000 ) ) ;
#7134=VERTEX_POINT ( 'NONE', #14561 ) ;
#7143=CIRCLE ( 'NONE', #12790, 2.649999999999992806 ) ;
#7154=SURFACE_SIDE_STYLE ('',( #2203 ) ) ;
#7155=EDGE_LOOP ( 'NONE', ( #4057, #6201, #8222, #6777 ) ) ;
#7157=CIRCLE ( 'NONE', #1718, 2.649999999999992806 ) ;
#7159=ORIENTED_EDGE ( 'NONE', *, *, #8812, .F. ) ;
#7167=DIRECTION ( 'NONE',  ( -0.000000000000000000, -1.000000000000000000, -0.000000000000000000 ) ) ;
#7175=CIRCLE ( 'NONE', #13868, 2.649999999999992806 ) ;
#7182=CIRCLE ( 'NONE', #15694, 75.00000000000001421 ) ;
#7185=FACE_BOUND ( 'NONE', #6555, .T. ) ;
#7224=CARTESIAN_POINT ( 'NONE',  ( -67.50000000000000000, 37.00000000000000000, 2.649999999999285816 ) ) ;
#7226=EDGE_CURVE ( 'NONE', #3694, #1275, #6168, .T. ) ;
#7245=DIRECTION ( 'NONE',  ( 0.8660254037844387076, -0.000000000000000000, -0.4999999999999998890 ) ) ;
#7260=CARTESIAN_POINT ( 'NONE',  ( 0.000000000000000000, 37.00000000000000000, 0.000000000000000000 ) ) ;
#7261=DIRECTION ( 'NONE',  ( 0.000000000000000000, 1.000000000000000000, 0.000000000000000000 ) ) ;
#7262=CARTESIAN_POINT ( 'NONE',  ( 2.143131898507869826E-15, 37.00000000000000000, -70.14999999999999147 ) ) ;
#7271=ORIENTED_EDGE ( 'NONE', *, *, #13132, .T. ) ;
#7316=DIRECTION ( 'NONE',  ( 0.000000000000000000, 0.000000000000000000, -1.000000000000000000 ) ) ;
#7326=EDGE_CURVE ( 'NONE', #946, #7457, #4830, .T. ) ;
#7333=DIRECTION ( 'NONE',  ( 0.000000000000000000, 1.000000000000000000, 0.000000000000000000 ) ) ;
#7346=ORIENTED_EDGE ( 'NONE', *, *, #8695, .T. ) ;
#7347=CARTESIAN_POINT ( 'NONE',  ( -21.01110699893041556, -1.230770033143087371E-15, -33.74230484541335073 ) ) ;
#7352=STYLED_ITEM ( 'NONE', ( #4566 ), #13909 ) ;
#7355=DIRECTION ( 'NONE',  ( -0.000000000000000000, -1.000000000000000000, -0.000000000000000000 ) ) ;
#7361=EDGE_CURVE ( 'NONE', #15747, #946, #8507, .T. ) ;
#7398=CARTESIAN_POINT ( 'NONE',  ( -21.01110699893060030, 0.000000000000000000, 36.39230484541324273 ) ) ;
#7399=EDGE_CURVE ( 'NONE', #8451, #2220, #8796, .T. ) ;
#7418=CIRCLE ( 'NONE', #452, 2.649999999999992806 ) ;
#7453=CIRCLE ( 'NONE', #15191, 32.00000000000000000 ) ;
#7457=VERTEX_POINT ( 'NONE', #13777 ) ;
#7480=AXIS2_PLACEMENT_3D ( 'NONE', #1134, #5016, #12197 ) ;
#7502=DIRECTION ( 'NONE',  ( -0.000000000000000000, -1.000000000000000000, -0.000000000000000000 ) ) ;
#7514=EDGE_LOOP ( 'NONE', ( #14519, #13033, #11454, #377 ) ) ;
#7615=AXIS2_PLACEMENT_3D ( 'NONE', #13623, #13295, #9670 ) ;
#7632=CARTESIAN_POINT ( 'NONE',  ( 0.000000000000000000, 40.00000000000000000, 0.000000000000000000 ) ) ;
#7666=DIRECTION ( 'NONE',  ( -0.000000000000000000, -1.000000000000000000, -0.000000000000000000 ) ) ;
#7699=CARTESIAN_POINT ( 'NONE',  ( -21.01110699893041556, 0.000000000000000000, -36.39230484541334221 ) ) ;
#7701=VERTEX_POINT ( 'NONE', #15572 ) ;
#7724=DIRECTION ( 'NONE',  ( -0.000000000000000000, -1.000000000000000000, -0.000000000000000000 ) ) ;
#7725=AXIS2_PLACEMENT_3D ( 'NONE', #5525, #11810, #2040 ) ;
#7728=EDGE_CURVE ( 'NONE', #9639, #14899, #11073, .T. ) ;
#7736=VECTOR ( 'NONE', #2235, 1000.000000000000000 ) ;
#7753=DIRECTION ( 'NONE',  ( -0.000000000000000000, -1.000000000000000000, -0.000000000000000000 ) ) ;
#7755=CARTESIAN_POINT ( 'NONE',  ( 0.000000000000000000, 40.00000000000000000, -60.00000000000000000 ) ) ;
#7766=ORIENTED_EDGE ( 'NONE', *, *, #2044, .F. ) ;
#7827=VECTOR ( 'NONE', #5434, 1000.000000000000000 ) ;
#7835=VERTEX_POINT ( 'NONE', #7083 ) ;
#7879=EDGE_CURVE ( 'NONE', #13350, #14899, #4650, .T. ) ;
#7882=STYLED_ITEM ( 'NONE', ( #5851 ), #9085 ) ;
#7893=ORIENTED_EDGE ( 'NONE', *, *, #10447, .T. ) ;
#7914=VERTEX_POINT ( 'NONE', #1494 ) ;
#7948=DIRECTION ( 'NONE',  ( 0.8660254037844387076, 0.000000000000000000, -0.4999999999999998890 ) ) ;
#7959=ORIENTED_EDGE ( 'NONE', *, *, #1161, .F. ) ;
#7960=CIRCLE ( 'NONE', #14924, 2.649999999999999467 ) ;
#7990=DIRECTION ( 'NONE',  ( 0.000000000000000000, 1.000000000000000000, 0.000000000000000000 ) ) ;
#8037=CARTESIAN_POINT ( 'NONE',  ( -28.86751345948129099, 1.999999999999998224, 18.00000000000000000 ) ) ;
#8048=CARTESIAN_POINT ( 'NONE',  ( 7.347880794884118356E-15, 37.00000000000000000, 60.00000000000000000 ) ) ;
#8052=CARTESIAN_POINT ( 'NONE',  ( -67.50000000000000000, 40.00000000000000000, -7.070249711157346244E-13 ) ) ;
#8054=EDGE_CURVE ( 'NONE', #14880, #9569, #11640, .T. ) ;
#8076=UNCERTAINTY_MEASURE_WITH_UNIT (LENGTH_MEASURE( 1.000000000000000082E-05 ), #8304, 'distance_accuracy_value', 'NONE');
#8101=AXIS2_PLACEMENT_3D ( 'NONE', #4209, #2996, #7948 ) ;
#8120=LINE ( 'NONE', #7224, #13804 ) ;
#8130=ORIENTED_EDGE ( 'NONE', *, *, #3235, .T. ) ;
#8146=CIRCLE ( 'NONE', #1662, 2.649999999999999467 ) ;
#8161=CARTESIAN_POINT ( 'NONE',  ( -1.154700538379235031, -20.00000000000000000, -34.00000000000000000 ) ) ;
#8176=DIRECTION ( 'NONE',  ( 0.000000000000000000, -0.000000000000000000, 1.000000000000000000 ) ) ;
#8197=ADVANCED_FACE ( 'NONE', ( #4385 ), #10612, .F. ) ;
#8215=( LENGTH_UNIT ( ) NAMED_UNIT ( * ) SI_UNIT ( .MILLI., .METRE. ) );
#8222=ORIENTED_EDGE ( 'NONE', *, *, #1971, .T. ) ;
#8282=VERTEX_POINT ( 'NONE', #15778 ) ;
#8304=( LENGTH_UNIT ( ) NAMED_UNIT ( * ) SI_UNIT ( .MILLI., .METRE. ) );
#8330=DIRECTION ( 'NONE',  ( 0.000000000000000000, 0.000000000000000000, 1.000000000000000000 ) ) ;
#8353=EDGE_LOOP ( 'NONE', ( #1671, #1056, #1281, #1007, #14840, #792 ) ) ;
#8355=CARTESIAN_POINT ( 'NONE',  ( -67.50000000000000000, 37.00000000000000000, -2.650000000000692690 ) ) ;
#8381=DIRECTION ( 'NONE',  ( -0.000000000000000000, -1.000000000000000000, -0.000000000000000000 ) ) ;
#8421=CARTESIAN_POINT ( 'NONE',  ( 42.02221399786069611, 0.000000000000000000, 2.650000000000100275 ) ) ;
#8425=DIRECTION ( 'NONE',  ( 0.000000000000000000, 0.000000000000000000, -1.000000000000000000 ) ) ;
#8432=DIRECTION ( 'NONE',  ( 0.000000000000000000, 0.000000000000000000, 1.000000000000000000 ) ) ;
#8433=ORIENTED_EDGE ( 'NONE', *, *, #15270, .F. ) ;
#8439=ORIENTED_EDGE ( 'NONE', *, *, #15270, .T. ) ;
#8445=CIRCLE ( 'NONE', #8688, 2.649999999999992806 ) ;
#8451=VERTEX_POINT ( 'NONE', #6474 ) ;
#8497=CARTESIAN_POINT ( 'NONE',  ( -28.86751345948196601, 1.999999999999998224, -75.00199999999976797 ) ) ;
#8507=CIRCLE ( 'NONE', #10572, 32.00000000000000000 ) ;
#8509=EDGE_CURVE ( 'NONE', #12023, #10516, #7182, .T. ) ;
#8516=EDGE_LOOP ( 'NONE', ( #989, #4682, #12253, #2075 ) ) ;
#8576=CARTESIAN_POINT ( 'NONE',  ( 2.467663300281918126E-15, 37.00000000000000000, -64.85000000000002274 ) ) ;
#8598=DIRECTION ( 'NONE',  ( 0.000000000000000000, 0.000000000000000000, 1.000000000000000000 ) ) ;
#8602=DIRECTION ( 'NONE',  ( 0.000000000000000000, 0.000000000000000000, -1.000000000000000000 ) ) ;
#8609=EDGE_CURVE ( 'NONE', #10728, #14880, #12575, .T. ) ;
#8624=ORIENTED_EDGE ( 'NONE', *, *, #8509, .F. ) ;
#8629=DIRECTION ( 'NONE',  ( 0.000000000000000000, 0.000000000000000000, -1.000000000000000000 ) ) ;
#8648=AXIS2_PLACEMENT_3D ( 'NONE', #7260, #7333, #3766 ) ;
#8662=EDGE_CURVE ( 'NONE', #12101, #7457, #731, .T. ) ;
#8685=ORIENTED_EDGE ( 'NONE', *, *, #5718, .T. ) ;
#8688=AXIS2_PLACEMENT_3D ( 'NONE', #9270, #4412, #9344 ) ;
#8695=EDGE_CURVE ( 'NONE', #4042, #8451, #6415, .T. ) ;
#8706=VECTOR ( 'NONE', #584, 1000.000000000000000 ) ;
#8748=ORIENTED_EDGE ( 'NONE', *, *, #7361, .T. ) ;
#8761=AXIS2_PLACEMENT_3D ( 'NONE', #12585, #2571, #13717 ) ;
#8788=EDGE_LOOP ( 'NONE', ( #111, #7959 ) ) ;
#8796=LINE ( 'NONE', #4004, #759 ) ;
#8804=VERTEX_POINT ( 'NONE', #4751 ) ;
#8812=EDGE_CURVE ( 'NONE', #1457, #138, #13875, .T. ) ;
#8815=FACE_OUTER_BOUND ( 'NONE', #1371, .T. ) ;
#8823=DIRECTION ( 'NONE',  ( -0.000000000000000000, -1.000000000000000000, -0.000000000000000000 ) ) ;
#8825=FACE_OUTER_BOUND ( 'NONE', #12173, .T. ) ;
#8837=CYLINDRICAL_SURFACE ( 'NONE', #3548, 31.99999999999999289 ) ;
#8849=AXIS2_PLACEMENT_3D ( 'NONE', #9214, #10658, #12907 ) ;
#8906=ORIENTED_EDGE ( 'NONE', *, *, #1811, .T. ) ;
#8923=EDGE_CURVE ( 'NONE', #6, #11302, #10289, .T. ) ;
#8936=AXIS2_PLACEMENT_3D ( 'NONE', #13960, #6540, #4187 ) ;
#8943=CARTESIAN_POINT ( 'NONE',  ( -28.86751345948112402, 0.000000000000000000, 18.00000000000026645 ) ) ;
#8996=EDGE_CURVE ( 'NONE', #15957, #2273, #6149, .T. ) ;
#9011=CARTESIAN_POINT ( 'NONE',  ( 7.347880794884118356E-15, 40.00000000000000000, 60.00000000000000000 ) ) ;
#9040=CYLINDRICAL_SURFACE ( 'NONE', #3282, 2.649999999999999467 ) ;
#9056=EDGE_LOOP ( 'NONE', ( #9339, #7001 ) ) ;
#9085=ADVANCED_BREP_SHAPE_REPRESENTATION ( '', ( #13909, #3223 ), #1673 ) ;
#9110=DIRECTION ( 'NONE',  ( 0.000000000000000000, 0.000000000000000000, 1.000000000000000000 ) ) ;
#9111=DIRECTION ( 'NONE',  ( -0.000000000000000000, -1.000000000000000000, -0.000000000000000000 ) ) ;
#9130=CARTESIAN_POINT ( 'NONE',  ( 7.102951435054648059E-15, 40.00000000000000000, 57.99999999999999289 ) ) ;
#9149=ORIENTED_EDGE ( 'NONE', *, *, #8609, .F. ) ;
#9153=CARTESIAN_POINT ( 'NONE',  ( -28.86751345948129099, -20.00000000000000000, 18.00000000000000000 ) ) ;
#9185=ORIENTED_EDGE ( 'NONE', *, *, #3035, .F. ) ;
#9190=AXIS2_PLACEMENT_3D ( 'NONE', #12921, #10674, #1854 ) ;
#9214=CARTESIAN_POINT ( 'NONE',  ( -67.50000000000000000, 37.00000000000000000, -7.070249711157346244E-13 ) ) ;
#9225=EDGE_LOOP ( 'NONE', ( #8685, #4323, #10005, #6012 ) ) ;
#9253=DIRECTION ( 'NONE',  ( 0.000000000000000000, 0.000000000000000000, 1.000000000000000000 ) ) ;
#9259=DIRECTION ( 'NONE',  ( 0.000000000000000000, 0.000000000000000000, -1.000000000000000000 ) ) ;
#9270=CARTESIAN_POINT ( 'NONE',  ( 42.02221399786069611, 2.000000000000000000, 1.075528555105620399E-13 ) ) ;
#9273=CIRCLE ( 'NONE', #13371, 2.649999999999985700 ) ;
#9276=CYLINDRICAL_SURFACE ( 'NONE', #6123, 32.00000000000000711 ) ;
#9302=DIRECTION ( 'NONE',  ( -1.734723475976807489E-15, 0.000000000000000000, 1.000000000000000000 ) ) ;
#9339=ORIENTED_EDGE ( 'NONE', *, *, #6047, .F. ) ;
#9344=DIRECTION ( 'NONE',  ( 0.000000000000000000, 0.000000000000000000, 1.000000000000000000 ) ) ;
#9361=VERTEX_POINT ( 'NONE', #15317 ) ;
#9391=CARTESIAN_POINT ( 'NONE',  ( -21.01110699893060030, 0.000000000000000000, 39.04230484541323420 ) ) ;
#9396=ORIENTED_EDGE ( 'NONE', *, *, #6366, .F. ) ;
#9414=CARTESIAN_POINT ( 'NONE',  ( -6.762176242291807225E-13, 40.00000000000000000, 70.14999999999930935 ) ) ;
#9493=ORIENTED_EDGE ( 'NONE', *, *, #11599, .F. ) ;
#9521=EDGE_CURVE ( 'NONE', #10516, #12023, #10024, .T. ) ;
#9529=CARTESIAN_POINT ( 'NONE',  ( -21.01110699893041556, 2.000000000000000000, -36.39230484541334221 ) ) ;
#9569=VERTEX_POINT ( 'NONE', #15056 ) ;
#9587=ORIENTED_EDGE ( 'NONE', *, *, #13550, .T. ) ;
#9598=EDGE_CURVE ( 'NONE', #8804, #6, #1120, .T. ) ;
#9609=CYLINDRICAL_SURFACE ( 'NONE', #11074, 2.649999999999999467 ) ;
#9618=VECTOR ( 'NONE', #1533, 1000.000000000000000 ) ;
#9625=DIRECTION ( 'NONE',  ( -0.000000000000000000, -1.000000000000000000, -0.000000000000000000 ) ) ;
#9639=VERTEX_POINT ( 'NONE', #10756 ) ;
#9645=FACE_OUTER_BOUND ( 'NONE', #2924, .T. ) ;
#9670=DIRECTION ( 'NONE',  ( 0.000000000000000000, 0.000000000000000000, -1.000000000000000000 ) ) ;
#9678=VERTEX_POINT ( 'NONE', #8576 ) ;
#9701=VECTOR ( 'NONE', #1992, 1000.000000000000000 ) ;
#9720=ADVANCED_FACE ( 'NONE', ( #2403 ), #9609, .F. ) ;
#9748=AXIS2_PLACEMENT_3D ( 'NONE', #11623, #5494, #4279 ) ;
#9749=CARTESIAN_POINT ( 'NONE',  ( -1.154700538379406893, 0.000000000000000000, -34.00000000000000711 ) ) ;
#9770=DIRECTION ( 'NONE',  ( 9.048317650695024227E-15, -0.000000000000000000, 1.000000000000000000 ) ) ;
#9785=DIRECTION ( 'NONE',  ( 0.000000000000000000, 0.000000000000000000, 1.000000000000000000 ) ) ;
#9789=ADVANCED_FACE ( 'NONE', ( #8815 ), #82, .T. ) ;
#9791=EDGE_CURVE ( 'NONE', #13808, #10876, #1531, .T. ) ;
#9807=ORIENTED_EDGE ( 'NONE', *, *, #15096, .F. ) ;
#9810=ORIENTED_EDGE ( 'NONE', *, *, #14190, .F. ) ;
#9814=DIRECTION ( 'NONE',  ( 0.000000000000000000, 1.000000000000000000, 0.000000000000000000 ) ) ;
#9823=CARTESIAN_POINT ( 'NONE',  ( 30.02221399786053624, -20.00000000000000000, 16.00000000000001421 ) ) ;
#9827=ORIENTED_EDGE ( 'NONE', *, *, #5943, .F. ) ;
#9852=EDGE_CURVE ( 'NONE', #9569, #865, #9273, .T. ) ;
#9864=ORIENTED_EDGE ( 'NONE', *, *, #1732, .F. ) ;
#9889=CARTESIAN_POINT ( 'NONE',  ( -6.765421556309547668E-13, 37.00000000000000000, 64.84999999999931219 ) ) ;
#9917=ORIENTED_EDGE ( 'NONE', *, *, #12980, .F. ) ;
#9940=DIRECTION ( 'NONE',  ( 0.000000000000000000, 0.000000000000000000, -1.000000000000000000 ) ) ;
#9972=CYLINDRICAL_SURFACE ( 'NONE', #12084, 2.649999999999992806 ) ;
#9988=EDGE_CURVE ( 'NONE', #10876, #13011, #2035, .T. ) ;
#10005=ORIENTED_EDGE ( 'NONE', *, *, #15096, .T. ) ;
#10024=CIRCLE ( 'NONE', #15164, 75.00000000000001421 ) ;
#10035=ORIENTED_EDGE ( 'NONE', *, *, #2834, .F. ) ;
#10043=EDGE_CURVE ( 'NONE', #1654, #9678, #15214, .T. ) ;
#10049=CARTESIAN_POINT ( 'NONE',  ( -28.86751345948129455, -20.00000000000000000, 49.99999999999999289 ) ) ;
#10072=DIRECTION ( 'NONE',  ( 0.000000000000000000, 0.000000000000000000, -1.000000000000000000 ) ) ;
#10098=ORIENTED_EDGE ( 'NONE', *, *, #2772, .F. ) ;
#10120=DIRECTION ( 'NONE',  ( 0.000000000000000000, 1.000000000000000000, 0.000000000000000000 ) ) ;
#10140=UNCERTAINTY_MEASURE_WITH_UNIT (LENGTH_MEASURE( 1.000000000000000082E-05 ), #15799, 'distance_accuracy_value', 'NONE');
#10154=VERTEX_POINT ( 'NONE', #15287 ) ;
#10189=FACE_BOUND ( 'NONE', #5994, .T. ) ;
#10201=DIRECTION ( 'NONE',  ( 0.000000000000000000, 1.000000000000000000, 0.000000000000000000 ) ) ;
#10223=DIRECTION ( 'NONE',  ( 0.000000000000000000, 0.000000000000000000, -1.000000000000000000 ) ) ;
#10240=DIRECTION ( 'NONE',  ( 0.000000000000000000, 0.000000000000000000, 1.000000000000000000 ) ) ;
#10251=CARTESIAN_POINT ( 'NONE',  ( 67.49999999999931788, 40.00000000000000000, 2.081668171172168513E-14 ) ) ;
#10254=LINE ( 'NONE', #9823, #4538 ) ;
#10259=ORIENTED_EDGE ( 'NONE', *, *, #8812, .T. ) ;
#10262=ORIENTED_EDGE ( 'NONE', *, *, #3035, .T. ) ;
#10277=DIRECTION ( 'NONE',  ( 0.000000000000000000, 1.000000000000000000, 0.000000000000000000 ) ) ;
#10287=VERTEX_POINT ( 'NONE', #7347 ) ;
#10289=CIRCLE ( 'NONE', #986, 2.649999999999985700 ) ;
#10318=ORIENTED_EDGE ( 'NONE', *, *, #8054, .F. ) ;
#10319=FACE_OUTER_BOUND ( 'NONE', #460, .T. ) ;
#10329=CARTESIAN_POINT ( 'NONE',  ( 42.02221399786069611, -1.230770033143087371E-15, 1.075528555105620399E-13 ) ) ;
#10340=ORIENTED_EDGE ( 'NONE', *, *, #7226, .F. ) ;
#10366=FACE_OUTER_BOUND ( 'NONE', #7514, .T. ) ;
#10395=EDGE_CURVE ( 'NONE', #739, #13808, #3087, .T. ) ;
#10418=CARTESIAN_POINT ( 'NONE',  ( 2.143131898507869826E-15, 37.00000000000000000, -67.50000000000000000 ) ) ;
#10424=DIRECTION ( 'NONE',  ( 0.000000000000000000, 1.000000000000000000, 0.000000000000000000 ) ) ;
#10437=CARTESIAN_POINT ( 'NONE',  ( -21.01110699893060030, -1.230770033143087371E-15, 36.39230484541324273 ) ) ;
#10444=AXIS2_PLACEMENT_3D ( 'NONE', #4513, #4367, #11696 ) ;
#10447=EDGE_CURVE ( 'NONE', #13350, #11846, #4110, .T. ) ;
#10462=CARTESIAN_POINT ( 'NONE',  ( 67.49999999999931788, 37.00000000000000000, 2.081668171172168513E-14 ) ) ;
#10501=CARTESIAN_POINT ( 'NONE',  ( 30.02221399786059663, 1.999999999999998224, -16.00000000000007461 ) ) ;
#10516=VERTEX_POINT ( 'NONE', #14343 ) ;
#10563=ORIENTED_EDGE ( 'NONE', *, *, #2734, .F. ) ;
#10572=AXIS2_PLACEMENT_3D ( 'NONE', #4908, #881, #5799 ) ;
#10592=DIRECTION ( 'NONE',  ( 0.000000000000000000, 0.000000000000000000, -1.000000000000000000 ) ) ;
#10612=CYLINDRICAL_SURFACE ( 'NONE', #976, 2.649999999999992806 ) ;
#10644=CARTESIAN_POINT ( 'NONE',  ( -6.762176242291807225E-13, 37.00000000000000000, 70.14999999999930935 ) ) ;
#10645=DIRECTION ( 'NONE',  ( -0.000000000000000000, -1.000000000000000000, -0.000000000000000000 ) ) ;
#10658=DIRECTION ( 'NONE',  ( -0.000000000000000000, -1.000000000000000000, -0.000000000000000000 ) ) ;
#10674=DIRECTION ( 'NONE',  ( -1.000000000000000000, 0.000000000000000000, 9.048317650695024227E-15 ) ) ;
#10713=MECHANICAL_DESIGN_GEOMETRIC_PRESENTATION_REPRESENTATION('',(#7882),#911);
#10716=LINE ( 'NONE', #2134, #3012 ) ;
#10717=CARTESIAN_POINT ( 'NONE',  ( 0.000000000000000000, 40.00000000000000000, 0.000000000000000000 ) ) ;
#10721=DIRECTION ( 'NONE',  ( -0.8660254037844408170, 0.000000000000000000, -0.4999999999999961142 ) ) ;
#10728=VERTEX_POINT ( 'NONE', #15228 ) ;
#10756=CARTESIAN_POINT ( 'NONE',  ( 7.102951435054648059E-15, 2.000000000000001776, 57.99999999999999289 ) ) ;
#10788=AXIS2_PLACEMENT_3D ( 'NONE', #4154, #132, #2617 ) ;
#10812=CYLINDRICAL_SURFACE ( 'NONE', #3500, 2.649999999999992806 ) ;
#10831=CARTESIAN_POINT ( 'NONE',  ( -67.50000000000000000, 37.00000000000000000, 2.649999999999278710 ) ) ;
#10841=ORIENTED_EDGE ( 'NONE', *, *, #9791, .F. ) ;
#10843=ORIENTED_EDGE ( 'NONE', *, *, #9852, .F. ) ;
#10857=EDGE_LOOP ( 'NONE', ( #267, #5933 ) ) ;
#10862=ORIENTED_EDGE ( 'NONE', *, *, #9598, .F. ) ;
#10876=VERTEX_POINT ( 'NONE', #8355 ) ;
#10902=ORIENTED_EDGE ( 'NONE', *, *, #6366, .T. ) ;
#10905=DIRECTION ( 'NONE',  ( -0.000000000000000000, -1.000000000000000000, -0.000000000000000000 ) ) ;
#10930=VECTOR ( 'NONE', #3286, 1000.000000000000000 ) ;
#10941=SURFACE_STYLE_FILL_AREA ( #1154 ) ;
#10991=ADVANCED_FACE ( 'NONE', ( #13564 ), #11004, .T. ) ;
#11004=CYLINDRICAL_SURFACE ( 'NONE', #7480, 32.00000000000000000 ) ;
#11006=ORIENTED_EDGE ( 'NONE', *, *, #12620, .T. ) ;
#11013=AXIS2_PLACEMENT_3D ( 'NONE', #11196, #382, #140 ) ;
#11018=SHAPE_REPRESENTATION_RELATIONSHIP ( 'NONE' , 'NONE' ,  #14733, #9085 ) ;
#11063=LINE ( 'NONE', #3695, #4803 ) ;
#11073=CIRCLE ( 'NONE', #11568, 57.99999999999999289 ) ;
#11074=AXIS2_PLACEMENT_3D ( 'NONE', #12111, #7355, #6148 ) ;
#11083=CARTESIAN_POINT ( 'NONE',  ( -28.86751345948129455, 0.000000000000000000, 49.99999999999999289 ) ) ;
#11091=DIRECTION ( 'NONE',  ( 0.000000000000000000, 1.000000000000000000, 0.000000000000000000 ) ) ;
#11177=CARTESIAN_POINT ( 'NONE',  ( 42.02221399786069611, 0.000000000000000000, 1.075528555105620399E-13 ) ) ;
#11182=DIRECTION ( 'NONE',  ( 0.000000000000000000, -1.000000000000000000, -0.000000000000000000 ) ) ;
#11187=CYLINDRICAL_SURFACE ( 'NONE', #10788, 2.649999999999999467 ) ;
#11196=CARTESIAN_POINT ( 'NONE',  ( 0.000000000000000000, 40.00000000000000000, 0.000000000000000000 ) ) ;
#11203=CIRCLE ( 'NONE', #14560, 2.649999999999985700 ) ;
#11276=EDGE_LOOP ( 'NONE', ( #675, #2560 ) ) ;
#11278=AXIS2_PLACEMENT_3D ( 'NONE', #10437, #14066, #12844 ) ;
#11286=FACE_OUTER_BOUND ( 'NONE', #7155, .T. ) ;
#11302=VERTEX_POINT ( 'NONE', #14468 ) ;
#11328=CARTESIAN_POINT ( 'NONE',  ( 0.000000000000000000, 37.00000000000000000, 0.000000000000000000 ) ) ;
#11332=DIRECTION ( 'NONE',  ( 0.000000000000000000, 1.000000000000000000, 0.000000000000000000 ) ) ;
#11357=ORIENTED_EDGE ( 'NONE', *, *, #12684, .T. ) ;
#11381=CARTESIAN_POINT ( 'NONE',  ( -21.01110699893060030, -1.230770033143087371E-15, 36.39230484541324273 ) ) ;
#11389=CARTESIAN_POINT ( 'NONE',  ( -67.50000000000000000, 40.00000000000000000, 2.649999999999285816 ) ) ;
#11400=ADVANCED_FACE ( 'NONE', ( #2096 ), #896, .F. ) ;
#11429=CIRCLE ( 'NONE', #4467, 31.99999999999999289 ) ;
#11432=ORIENTED_EDGE ( 'NONE', *, *, #6597, .F. ) ;
#11447=ORIENTED_EDGE ( 'NONE', *, *, #9598, .T. ) ;
#11454=ORIENTED_EDGE ( 'NONE', *, *, #7399, .T. ) ;
#11476=COLOUR_RGB ( '', 0.66274510, 0.83137255, 0.94901961) ;
#11490=DIRECTION ( 'NONE',  ( 0.000000000000000000, 1.000000000000000000, 0.000000000000000000 ) ) ;
#11497=CARTESIAN_POINT ( 'NONE',  ( 30.02221399786054334, 0.000000000000000000, 16.00000000000000355 ) ) ;
#11515=DIRECTION ( 'NONE',  ( 0.000000000000000000, 0.000000000000000000, -1.000000000000000000 ) ) ;
#11516=CLOSED_SHELL ( 'NONE', ( #1235, #6803, #14781, #3254, #3665, #9720, #1555, #364, #4932, #9789, #15030, #12248, #1933, #833, #7025, #3924, #10991, #4704, #3755, #13412, #956, #3279, #11400, #12324, #4545, #8197, #5880, #12011, #21, #2083 ) ) ;
#11517=CARTESIAN_POINT ( 'NONE',  ( -6.765421556309547668E-13, 37.00000000000000000, 67.49999999999930367 ) ) ;
#11559=EDGE_LOOP ( 'NONE', ( #7159, #2986 ) ) ;
#11561=LINE ( 'NONE', #515, #7827 ) ;
#11563=AXIS2_PLACEMENT_3D ( 'NONE', #15796, #14567, #13420 ) ;
#11568=AXIS2_PLACEMENT_3D ( 'NONE', #15500, #14201, #5631 ) ;
#11599=EDGE_CURVE ( 'NONE', #946, #4042, #2250, .T. ) ;
#11616=EDGE_CURVE ( 'NONE', #10728, #865, #1044, .T. ) ;
#11623=CARTESIAN_POINT ( 'NONE',  ( -28.86751345948126257, 0.000000000000000000, -50.00000000000000711 ) ) ;
#11640=LINE ( 'NONE', #9391, #13369 ) ;
#11653=CYLINDRICAL_SURFACE ( 'NONE', #7725, 57.99999999999999289 ) ;
#11691=CARTESIAN_POINT ( 'NONE',  ( -67.50000000000000000, 37.00000000000000000, -7.070249711157346244E-13 ) ) ;
#11696=DIRECTION ( 'NONE',  ( 0.000000000000000000, 0.000000000000000000, -1.000000000000000000 ) ) ;
#11725=ORIENTED_EDGE ( 'NONE', *, *, #9988, .T. ) ;
#11763=EDGE_LOOP ( 'NONE', ( #9810, #15059 ) ) ;
#11810=DIRECTION ( 'NONE',  ( -0.000000000000000000, -1.000000000000000000, -0.000000000000000000 ) ) ;
#11835=FACE_BOUND ( 'NONE', #11559, .T. ) ;
#11840=CARTESIAN_POINT ( 'NONE',  ( 42.02221399786069611, -1.230770033143087371E-15, 1.075528555105620399E-13 ) ) ;
#11846=VERTEX_POINT ( 'NONE', #9130 ) ;
#11859=CARTESIAN_POINT ( 'NONE',  ( -6.765421556309547668E-13, 37.00000000000000000, 67.49999999999930367 ) ) ;
#11871=VERTEX_POINT ( 'NONE', #10501 ) ;
#11897=CARTESIAN_POINT ( 'NONE',  ( 0.000000000000000000, 0.000000000000000000, 0.000000000000000000 ) ) ;
#11910=FACE_BOUND ( 'NONE', #15705, .T. ) ;
#11929=CARTESIAN_POINT ( 'NONE',  ( -28.86751345948126612, -20.00000000000000000, -18.00000000000000711 ) ) ;
#11937=CARTESIAN_POINT ( 'NONE',  ( 0.000000000000000000, 0.000000000000000000, 0.000000000000000000 ) ) ;
#11958=ORIENTED_EDGE ( 'NONE', *, *, #86, .F. ) ;
#11972=DIRECTION ( 'NONE',  ( 0.000000000000000000, 0.000000000000000000, 1.000000000000000000 ) ) ;
#11993=CARTESIAN_POINT ( 'NONE',  ( 2.467663300281917732E-15, 37.00000000000000000, -64.85000000000000853 ) ) ;
#11994=ORIENTED_EDGE ( 'NONE', *, *, #7326, .T. ) ;
#11998=VECTOR ( 'NONE', #5076, 1000.000000000000000 ) ;
#12002=VECTOR ( 'NONE', #9770, 1000.000000000000000 ) ;
#12011=ADVANCED_FACE ( 'NONE', ( #5878 ), #10812, .F. ) ;
#12023=VERTEX_POINT ( 'NONE', #6038 ) ;
#12033=AXIS2_PLACEMENT_3D ( 'NONE', #4889, #9814, #14743 ) ;
#12055=FILL_AREA_STYLE_COLOUR ( '', #11476 ) ;
#12058=ORIENTED_EDGE ( 'NONE', *, *, #1161, .T. ) ;
#12084=AXIS2_PLACEMENT_3D ( 'NONE', #11177, #5282, #14092 ) ;
#12101=VERTEX_POINT ( 'NONE', #9749 ) ;
#12111=CARTESIAN_POINT ( 'NONE',  ( -6.765421556309547668E-13, 37.00000000000000000, 67.49999999999930367 ) ) ;
#12146=FACE_OUTER_BOUND ( 'NONE', #15023, .T. ) ;
#12173=EDGE_LOOP ( 'NONE', ( #13706, #10262, #1150, #4868 ) ) ;
#12179=LINE ( 'NONE', #8421, #4017 ) ;
#12197=DIRECTION ( 'NONE',  ( 0.000000000000000000, 0.000000000000000000, 1.000000000000000000 ) ) ;
#12198=ORIENTED_EDGE ( 'NONE', *, *, #10043, .T. ) ;
#12239=CIRCLE ( 'NONE', #5291, 2.649999999999992806 ) ;
#12248=ADVANCED_FACE ( 'NONE', ( #2793 ), #6282, .T. ) ;
#12250=ORIENTED_EDGE ( 'NONE', *, *, #10043, .F. ) ;
#12253=ORIENTED_EDGE ( 'NONE', *, *, #9852, .T. ) ;
#12261=VECTOR ( 'NONE', #12471, 1000.000000000000000 ) ;
#12264=CARTESIAN_POINT ( 'NONE',  ( 0.000000000000000000, 37.00000000000000000, -60.00000000000000000 ) ) ;
#12324=ADVANCED_FACE ( 'NONE', ( #3120 ), #15253, .F. ) ;
#12339=VECTOR ( 'NONE', #12388, 1000.000000000000000 ) ;
#12349=AXIS2_PLACEMENT_3D ( 'NONE', #10418, #646, #10592 ) ;
#12379=DIRECTION ( 'NONE',  ( 0.000000000000000000, 0.000000000000000000, 1.000000000000000000 ) ) ;
#12388=DIRECTION ( 'NONE',  ( -0.000000000000000000, -1.000000000000000000, -0.000000000000000000 ) ) ;
#12399=EDGE_LOOP ( 'NONE', ( #15802, #14800, #8439, #13228 ) ) ;
#12427=CARTESIAN_POINT ( 'NONE',  ( -67.50000000000000000, 37.00000000000000000, -7.070249711157346244E-13 ) ) ;
#12437=EDGE_CURVE ( 'NONE', #9361, #8804, #8445, .T. ) ;
#12471=DIRECTION ( 'NONE',  ( 9.048317650695024227E-15, -0.000000000000000000, 1.000000000000000000 ) ) ;
#12472=ORIENTED_EDGE ( 'NONE', *, *, #13615, .T. ) ;
#12485=DIRECTION ( 'NONE',  ( -0.000000000000000000, -1.000000000000000000, -0.000000000000000000 ) ) ;
#12560=DIRECTION ( 'NONE',  ( 0.000000000000000000, 1.000000000000000000, 0.000000000000000000 ) ) ;
#12565=DIRECTION ( 'NONE',  ( 0.000000000000000000, 0.000000000000000000, -1.000000000000000000 ) ) ;
#12567=DIRECTION ( 'NONE',  ( 0.8660254037844387076, -0.000000000000000000, -0.4999999999999998890 ) ) ;
#12575=CIRCLE ( 'NONE', #5626, 2.649999999999992806 ) ;
#12583=CIRCLE ( 'NONE', #15455, 32.00000000000000000 ) ;
#12585=CARTESIAN_POINT ( 'NONE',  ( 0.000000000000000000, 40.00000000000000000, 0.000000000000000000 ) ) ;
#12620=EDGE_CURVE ( 'NONE', #14899, #9639, #1713, .T. ) ;
#12684=EDGE_CURVE ( 'NONE', #8282, #10516, #15216, .T. ) ;
#12699=EDGE_CURVE ( 'NONE', #4101, #4042, #6560, .T. ) ;
#12711=CARTESIAN_POINT ( 'NONE',  ( -6.765421556309547668E-13, 37.00000000000000000, 64.84999999999932641 ) ) ;
#12723=EDGE_CURVE ( 'NONE', #865, #9569, #14122, .T. ) ;
#12784=ORIENTED_EDGE ( 'NONE', *, *, #14213, .T. ) ;
#12790=AXIS2_PLACEMENT_3D ( 'NONE', #1471, #11332, #15133 ) ;
#12800=AXIS2_PLACEMENT_3D ( 'NONE', #13749, #11490, #12379 ) ;
#12806=CARTESIAN_POINT ( 'NONE',  ( -21.01110699893041556, 0.000000000000000000, -33.74230484541335073 ) ) ;
#12844=DIRECTION ( 'NONE',  ( 0.000000000000000000, 0.000000000000000000, -1.000000000000000000 ) ) ;
#12864=VERTEX_POINT ( 'NONE', #15458 ) ;
#12907=DIRECTION ( 'NONE',  ( 0.000000000000000000, 0.000000000000000000, -1.000000000000000000 ) ) ;
#12921=CARTESIAN_POINT ( 'NONE',  ( -28.86751345948196601, 1.999999999999998224, -75.00199999999976797 ) ) ;
#12959=VECTOR ( 'NONE', #4167, 1000.000000000000000 ) ;
#12980=EDGE_CURVE ( 'NONE', #9361, #11302, #12179, .T. ) ;
#12989=EDGE_LOOP ( 'NONE', ( #14033, #9396 ) ) ;
#12994=ORIENTED_EDGE ( 'NONE', *, *, #5718, .F. ) ;
#13011=VERTEX_POINT ( 'NONE', #10831 ) ;
#13033=ORIENTED_EDGE ( 'NONE', *, *, #15137, .F. ) ;
#13053=CARTESIAN_POINT ( 'NONE',  ( -21.01110699893041556, 0.000000000000000000, -39.04230484541333368 ) ) ;
#13062=LINE ( 'NONE', #8161, #1931 ) ;
#13090=APPLICATION_CONTEXT ( 'automotive_design' ) ;
#13101=AXIS2_PLACEMENT_3D ( 'NONE', #6848, #5780, #10721 ) ;
#13115=( NAMED_UNIT ( * ) PLANE_ANGLE_UNIT ( ) SI_UNIT ( $, .RADIAN. ) );
#13132=EDGE_CURVE ( 'NONE', #1169, #15878, #2685, .T. ) ;
#13157=DIRECTION ( 'NONE',  ( -0.000000000000000000, -1.000000000000000000, -0.000000000000000000 ) ) ;
#13221=CIRCLE ( 'NONE', #14045, 2.649999999999992806 ) ;
#13224=EDGE_LOOP ( 'NONE', ( #10098, #3112 ) ) ;
#13228=ORIENTED_EDGE ( 'NONE', *, *, #13327, .F. ) ;
#13257=ORIENTED_EDGE ( 'NONE', *, *, #7728, .F. ) ;
#13288=VECTOR ( 'NONE', #5978, 1000.000000000000000 ) ;
#13295=DIRECTION ( 'NONE',  ( -0.000000000000000000, -1.000000000000000000, -0.000000000000000000 ) ) ;
#13327=EDGE_CURVE ( 'NONE', #12101, #15747, #13062, .T. ) ;
#13350=VERTEX_POINT ( 'NONE', #2078 ) ;
#13354=( NAMED_UNIT ( * ) SI_UNIT ( $, .STERADIAN. ) SOLID_ANGLE_UNIT ( ) );
#13359=AXIS2_PLACEMENT_3D ( 'NONE', #631, #3200, #3361 ) ;
#13369=VECTOR ( 'NONE', #6808, 1000.000000000000000 ) ;
#13371=AXIS2_PLACEMENT_3D ( 'NONE', #11381, #3705, #6305 ) ;
#13388=FACE_BOUND ( 'NONE', #642, .T. ) ;
#13389=ORIENTED_EDGE ( 'NONE', *, *, #10395, .T. ) ;
#13399=CARTESIAN_POINT ( 'NONE',  ( -6.762176242291807225E-13, 37.00000000000000000, 70.14999999999929514 ) ) ;
#13412=ADVANCED_FACE ( 'NONE', ( #7185, #3608, #1263, #14601, #14522, #3442 ), #15903, .F. ) ;
#13420=DIRECTION ( 'NONE',  ( 0.000000000000000000, 0.000000000000000000, 1.000000000000000000 ) ) ;
#13423=FACE_OUTER_BOUND ( 'NONE', #2596, .T. ) ;
#13430=LINE ( 'NONE', #9889, #81 ) ;
#13494=EDGE_LOOP ( 'NONE', ( #5619, #1387, #5478, #5342 ) ) ;
#13519=EDGE_CURVE ( 'NONE', #11302, #6, #387, .T. ) ;
#13536=AXIS2_PLACEMENT_3D ( 'NONE', #7699, #5098, #9940 ) ;
#13537=DIRECTION ( 'NONE',  ( -0.8660254037844408170, -0.000000000000000000, -0.4999999999999961142 ) ) ;
#13549=CARTESIAN_POINT ( 'NONE',  ( -67.50000000000000000, 37.00000000000000000, -2.650000000000699352 ) ) ;
#13550=EDGE_CURVE ( 'NONE', #11846, #9639, #13614, .T. ) ;
#13552=DIRECTION ( 'NONE',  ( -0.000000000000000000, -1.000000000000000000, -0.000000000000000000 ) ) ;
#13564=FACE_OUTER_BOUND ( 'NONE', #14796, .T. ) ;
#13614=LINE ( 'NONE', #15082, #660 ) ;
#13615=EDGE_CURVE ( 'NONE', #7701, #7037, #8146, .T. ) ;
#13623=CARTESIAN_POINT ( 'NONE',  ( -21.01110699893041556, -1.230770033143087371E-15, -36.39230484541334221 ) ) ;
#13624=VECTOR ( 'NONE', #8381, 1000.000000000000000 ) ;
#13634=AXIS2_PLACEMENT_3D ( 'NONE', #11328, #10120, #5265 ) ;
#13688=LINE ( 'NONE', #15003, #12261 ) ;
#13706=ORIENTED_EDGE ( 'NONE', *, *, #2772, .T. ) ;
#13717=DIRECTION ( 'NONE',  ( 0.000000000000000000, 0.000000000000000000, -1.000000000000000000 ) ) ;
#13734=ORIENTED_EDGE ( 'NONE', *, *, #1383, .T. ) ;
#13744=CARTESIAN_POINT ( 'NONE',  ( 57.73502691896258199, 1.999999999999998224, 2.081668171172168513E-14 ) ) ;
#13749=CARTESIAN_POINT ( 'NONE',  ( 0.000000000000000000, 0.000000000000000000, 0.000000000000000000 ) ) ;
#13751=EDGE_LOOP ( 'NONE', ( #3079, #13992, #56, #10862 ) ) ;
#13771=DIRECTION ( 'NONE',  ( 0.000000000000000000, 1.000000000000000000, 0.000000000000000000 ) ) ;
#13777=CARTESIAN_POINT ( 'NONE',  ( -28.86751345948126257, 0.000000000000000000, -18.00000000000001066 ) ) ;
#13792=ORIENTED_EDGE ( 'NONE', *, *, #12699, .T. ) ;
#13804=VECTOR ( 'NONE', #9625, 1000.000000000000000 ) ;
#13808=VERTEX_POINT ( 'NONE', #14020 ) ;
#13849=LINE ( 'NONE', #13928, #101 ) ;
#13868=AXIS2_PLACEMENT_3D ( 'NONE', #14922, #5292, #10072 ) ;
#13875=CIRCLE ( 'NONE', #5887, 2.649999999999992806 ) ;
#13909=MANIFOLD_SOLID_BREP ( 'CirPattern3', #11516 ) ;
#13917=ORIENTED_EDGE ( 'NONE', *, *, #9791, .T. ) ;
#13928=CARTESIAN_POINT ( 'NONE',  ( 30.02221399786055755, -20.00000000000000000, -15.99999999999999645 ) ) ;
#13941=CARTESIAN_POINT ( 'NONE',  ( 2.143131898507869826E-15, 40.00000000000000000, -67.50000000000000000 ) ) ;
#13943=LINE ( 'NONE', #7755, #12959 ) ;
#13954=ORIENTED_EDGE ( 'NONE', *, *, #15710, .T. ) ;
#13960=CARTESIAN_POINT ( 'NONE',  ( -6.765421556309547668E-13, 37.00000000000000000, 67.49999999999930367 ) ) ;
#13989=ORIENTED_EDGE ( 'NONE', *, *, #1971, .F. ) ;
#13992=ORIENTED_EDGE ( 'NONE', *, *, #12980, .T. ) ;
#13994=LINE ( 'NONE', #9011, #3527 ) ;
#14007=CARTESIAN_POINT ( 'NONE',  ( 79.38739406438118351, 0.000000000000000000, 12.50099999999964417 ) ) ;
#14020=CARTESIAN_POINT ( 'NONE',  ( -67.50000000000000000, 40.00000000000000000, -2.650000000000699352 ) ) ;
#14033=ORIENTED_EDGE ( 'NONE', *, *, #10447, .F. ) ;
#14045=AXIS2_PLACEMENT_3D ( 'NONE', #9529, #3145, #8330 ) ;
#14055=DIRECTION ( 'NONE',  ( -1.734723475976807489E-15, 0.000000000000000000, 1.000000000000000000 ) ) ;
#14066=DIRECTION ( 'NONE',  ( -0.000000000000000000, -1.000000000000000000, -0.000000000000000000 ) ) ;
#14073=CARTESIAN_POINT ( 'NONE',  ( 30.02221399786053624, 1.999999999999998224, 16.00000000000001421 ) ) ;
#14092=DIRECTION ( 'NONE',  ( 0.000000000000000000, 0.000000000000000000, -1.000000000000000000 ) ) ;
#14093=DIRECTION ( 'NONE',  ( 0.000000000000000000, 1.000000000000000000, 0.000000000000000000 ) ) ;
#14122=CIRCLE ( 'NONE', #11278, 2.649999999999985700 ) ;
#14143=CARTESIAN_POINT ( 'NONE',  ( 0.000000000000000000, 40.00000000000000000, 0.000000000000000000 ) ) ;
#14152=AXIS2_PLACEMENT_3D ( 'NONE', #825, #15780, #8432 ) ;
#14180=CARTESIAN_POINT ( 'NONE',  ( 2.143131898507869826E-15, 40.00000000000000000, -70.15000000000000568 ) ) ;
#14189=FILL_AREA_STYLE ('',( #12055 ) ) ;
#14190=EDGE_CURVE ( 'NONE', #8804, #9361, #12239, .T. ) ;
#14201=DIRECTION ( 'NONE',  ( 0.000000000000000000, 1.000000000000000000, 0.000000000000000000 ) ) ;
#14213=EDGE_CURVE ( 'NONE', #739, #13011, #8120, .T. ) ;
#14224=CARTESIAN_POINT ( 'NONE',  ( -28.86751345948129455, 1.999999999999998224, 49.99999999999999289 ) ) ;
#14273=DIRECTION ( 'NONE',  ( 0.000000000000000000, 0.000000000000000000, -1.000000000000000000 ) ) ;
#14325=ORIENTED_EDGE ( 'NONE', *, *, #13327, .T. ) ;
#14343=CARTESIAN_POINT ( 'NONE',  ( 9.184850993605150311E-15, 40.00000000000000000, -75.00000000000001421 ) ) ;
#14346=CARTESIAN_POINT ( 'NONE',  ( -21.01110699893041556, -1.230770033143087371E-15, -39.04230484541333368 ) ) ;
#14354=FACE_BOUND ( 'NONE', #3333, .T. ) ;
#14380=DIRECTION ( 'NONE',  ( 0.000000000000000000, 0.000000000000000000, 1.000000000000000000 ) ) ;
#14387=AXIS2_PLACEMENT_3D ( 'NONE', #368, #5283, #10223 ) ;
#14421=DIRECTION ( 'NONE',  ( 0.000000000000000000, 0.000000000000000000, 1.000000000000000000 ) ) ;
#14447=ORIENTED_EDGE ( 'NONE', *, *, #83, .F. ) ;
#14468=CARTESIAN_POINT ( 'NONE',  ( 42.02221399786069611, -1.230770033143087371E-15, 2.650000000000093170 ) ) ;
#14475=EDGE_CURVE ( 'NONE', #12864, #12101, #5140, .T. ) ;
#14509=LINE ( 'NONE', #5949, #12339 ) ;
#14519=ORIENTED_EDGE ( 'NONE', *, *, #4767, .F. ) ;
#14522=FACE_BOUND ( 'NONE', #3894, .T. ) ;
#14532=DIRECTION ( 'NONE',  ( 0.000000000000000000, 0.000000000000000000, -1.000000000000000000 ) ) ;
#14542=ORIENTED_EDGE ( 'NONE', *, *, #14213, .F. ) ;
#14550=DIRECTION ( 'NONE',  ( 0.000000000000000000, 0.000000000000000000, -1.000000000000000000 ) ) ;
#14560=AXIS2_PLACEMENT_3D ( 'NONE', #11859, #6958, #14532 ) ;
#14561=CARTESIAN_POINT ( 'NONE',  ( -21.01110699893041556, 2.000000000000000000, -39.04230484541333368 ) ) ;
#14567=DIRECTION ( 'NONE',  ( 0.000000000000000000, 1.000000000000000000, 0.000000000000000000 ) ) ;
#14601=FACE_BOUND ( 'NONE', #8788, .T. ) ;
#14633=CIRCLE ( 'NONE', #12033, 75.00000000000001421 ) ;
#14640=DIRECTION ( 'NONE',  ( -0.000000000000000000, -1.000000000000000000, -0.000000000000000000 ) ) ;
#14667=CYLINDRICAL_SURFACE ( 'NONE', #14387, 57.99999999999999289 ) ;
#14705=CARTESIAN_POINT ( 'NONE',  ( -21.01110699893060030, 0.000000000000000000, 33.74230484541324415 ) ) ;
#14733=SHAPE_REPRESENTATION ( 'Circular Main Body Shell', ( #3223 ), #1673 ) ;
#14743=DIRECTION ( 'NONE',  ( 0.000000000000000000, 0.000000000000000000, 1.000000000000000000 ) ) ;
#14752=DIRECTION ( 'NONE',  ( 0.000000000000000000, 1.000000000000000000, -0.000000000000000000 ) ) ;
#14754=ORIENTED_EDGE ( 'NONE', *, *, #1732, .T. ) ;
#14781=ADVANCED_FACE ( 'NONE', ( #8825 ), #19, .F. ) ;
#14782=AXIS2_PLACEMENT_3D ( 'NONE', #237, #5155, #15012 ) ;
#14786=DIRECTION ( 'NONE',  ( -0.000000000000000000, -1.000000000000000000, -0.000000000000000000 ) ) ;
#14796=EDGE_LOOP ( 'NONE', ( #11432, #13954, #2745, #5893 ) ) ;
#14800=ORIENTED_EDGE ( 'NONE', *, *, #3480, .F. ) ;
#14840=ORIENTED_EDGE ( 'NONE', *, *, #688, .T. ) ;
#14880=VERTEX_POINT ( 'NONE', #5341 ) ;
#14899=VERTEX_POINT ( 'NONE', #1779 ) ;
#14907=EDGE_LOOP ( 'NONE', ( #6051, #4038, #3391, #2174 ) ) ;
#14922=CARTESIAN_POINT ( 'NONE',  ( -21.01110699893041556, -1.230770033143087371E-15, -36.39230484541334221 ) ) ;
#14924=AXIS2_PLACEMENT_3D ( 'NONE', #5916, #7132, #9785 ) ;
#14987=ORIENTED_EDGE ( 'NONE', *, *, #5391, .F. ) ;
#15003=CARTESIAN_POINT ( 'NONE',  ( -28.86751345948196601, 0.000000000000000000, -75.00199999999976797 ) ) ;
#15012=DIRECTION ( 'NONE',  ( 0.000000000000000000, 0.000000000000000000, 1.000000000000000000 ) ) ;
#15023=EDGE_LOOP ( 'NONE', ( #10318, #5855, #5876, #4579 ) ) ;
#15029=AXIS2_PLACEMENT_3D ( 'NONE', #7398, #14640, #4890 ) ;
#15030=ADVANCED_FACE ( 'NONE', ( #4519, #5731, #4444, #2164, #13388 ), #3227, .F. ) ;
#15045=ORIENTED_EDGE ( 'NONE', *, *, #12699, .F. ) ;
#15056=CARTESIAN_POINT ( 'NONE',  ( -21.01110699893060030, -1.230770033143087371E-15, 39.04230484541322710 ) ) ;
#15059=ORIENTED_EDGE ( 'NONE', *, *, #12437, .F. ) ;
#15061=CARTESIAN_POINT ( 'NONE',  ( 67.49999999999931788, 37.00000000000000000, -2.649999999999971934 ) ) ;
#15080=CARTESIAN_POINT ( 'NONE',  ( 0.000000000000000000, 37.00000000000000000, 0.000000000000000000 ) ) ;
#15082=CARTESIAN_POINT ( 'NONE',  ( 7.102951435054648059E-15, 40.00000000000000000, 57.99999999999999289 ) ) ;
#15096=EDGE_CURVE ( 'NONE', #9678, #1654, #674, .T. ) ;
#15133=DIRECTION ( 'NONE',  ( 0.000000000000000000, 0.000000000000000000, 1.000000000000000000 ) ) ;
#15137=EDGE_CURVE ( 'NONE', #8451, #6399, #6378, .T. ) ;
#15163=EDGE_LOOP ( 'NONE', ( #7766, #10563 ) ) ;
#15164=AXIS2_PLACEMENT_3D ( 'NONE', #7632, #33, #8598 ) ;
#15181=ORIENTED_EDGE ( 'NONE', *, *, #86, .T. ) ;
#15191=AXIS2_PLACEMENT_3D ( 'NONE', #5982, #10905, #2484 ) ;
#15205=DIRECTION ( 'NONE',  ( 0.000000000000000000, -0.000000000000000000, 1.000000000000000000 ) ) ;
#15214=CIRCLE ( 'NONE', #12349, 2.649999999999985700 ) ;
#15216=LINE ( 'NONE', #2668, #2234 ) ;
#15228=CARTESIAN_POINT ( 'NONE',  ( -21.01110699893060030, 2.000000000000000000, 33.74230484541324415 ) ) ;
#15253=CYLINDRICAL_SURFACE ( 'NONE', #187, 2.649999999999992806 ) ;
#15270=EDGE_CURVE ( 'NONE', #11871, #15747, #11063, .T. ) ;
#15287=CARTESIAN_POINT ( 'NONE',  ( 0.000000000000000000, 0.000000000000000000, -60.00000000000000000 ) ) ;
#15296=PLANE ( 'NONE',  #8101 ) ;
#15317=CARTESIAN_POINT ( 'NONE',  ( 42.02221399786069611, 2.000000000000000000, 2.650000000000100275 ) ) ;
#15367=COLOUR_RGB ( '', 0.66274510, 0.83137255, 0.94901961) ;
#15396=FACE_OUTER_BOUND ( 'NONE', #1851, .T. ) ;
#15403=EDGE_LOOP ( 'NONE', ( #4106, #4712, #14754, #3100 ) ) ;
#15416=DIRECTION ( 'NONE',  ( 0.000000000000000000, 1.000000000000000000, 0.000000000000000000 ) ) ;
#15455=AXIS2_PLACEMENT_3D ( 'NONE', #13744, #2676, #6418 ) ;
#15458=CARTESIAN_POINT ( 'NONE',  ( 30.02221399786055400, 0.000000000000000000, -15.99999999999999645 ) ) ;
#15495=EDGE_CURVE ( 'NONE', #7134, #434, #6943, .T. ) ;
#15500=CARTESIAN_POINT ( 'NONE',  ( 0.000000000000000000, 2.000000000000001776, 0.000000000000000000 ) ) ;
#15530=EDGE_CURVE ( 'NONE', #7701, #9678, #7092, .T. ) ;
#15540=CARTESIAN_POINT ( 'NONE',  ( 67.49999999999931788, 37.00000000000000000, 2.081668171172168513E-14 ) ) ;
#15569=CARTESIAN_POINT ( 'NONE',  ( -67.50000000000000000, 37.00000000000000000, -7.070249711157346244E-13 ) ) ;
#15572=CARTESIAN_POINT ( 'NONE',  ( 2.467663300281916943E-15, 40.00000000000000000, -64.85000000000000853 ) ) ;
#15574=CYLINDRICAL_SURFACE ( 'NONE', #13359, 2.649999999999999467 ) ;
#15616=EDGE_CURVE ( 'NONE', #7457, #4101, #13688, .T. ) ;
#15637=ORIENTED_EDGE ( 'NONE', *, *, #226, .T. ) ;
#15648=FILL_AREA_STYLE_COLOUR ( '', #15367 ) ;
#15694=AXIS2_PLACEMENT_3D ( 'NONE', #14143, #573, #14380 ) ;
#15705=EDGE_LOOP ( 'NONE', ( #5712, #5055 ) ) ;
#15710=EDGE_CURVE ( 'NONE', #5167, #2220, #10254, .T. ) ;
#15735=VECTOR ( 'NONE', #406, 1000.000000000000000 ) ;
#15747=VERTEX_POINT ( 'NONE', #4326 ) ;
#15778=CARTESIAN_POINT ( 'NONE',  ( 9.184850993605150311E-15, 37.00000000000000000, -75.00000000000001421 ) ) ;
#15780=DIRECTION ( 'NONE',  ( 0.000000000000000000, 1.000000000000000000, 0.000000000000000000 ) ) ;
#15796=CARTESIAN_POINT ( 'NONE',  ( 0.000000000000000000, 40.00000000000000000, 0.000000000000000000 ) ) ;
#15799=( LENGTH_UNIT ( ) NAMED_UNIT ( * ) SI_UNIT ( .MILLI., .METRE. ) );
#15802=ORIENTED_EDGE ( 'NONE', *, *, #14475, .F. ) ;
#15876=CYLINDRICAL_SURFACE ( 'NONE', #6100, 2.649999999999992806 ) ;
#15878=VERTEX_POINT ( 'NONE', #12711 ) ;
#15903=PLANE ( 'NONE',  #8648 ) ;
#15945=DIRECTION ( 'NONE',  ( 0.000000000000000000, 0.000000000000000000, 1.000000000000000000 ) ) ;
#15957=VERTEX_POINT ( 'NONE', #9414 ) ;
ENDSEC;
END-ISO-10303-21;
